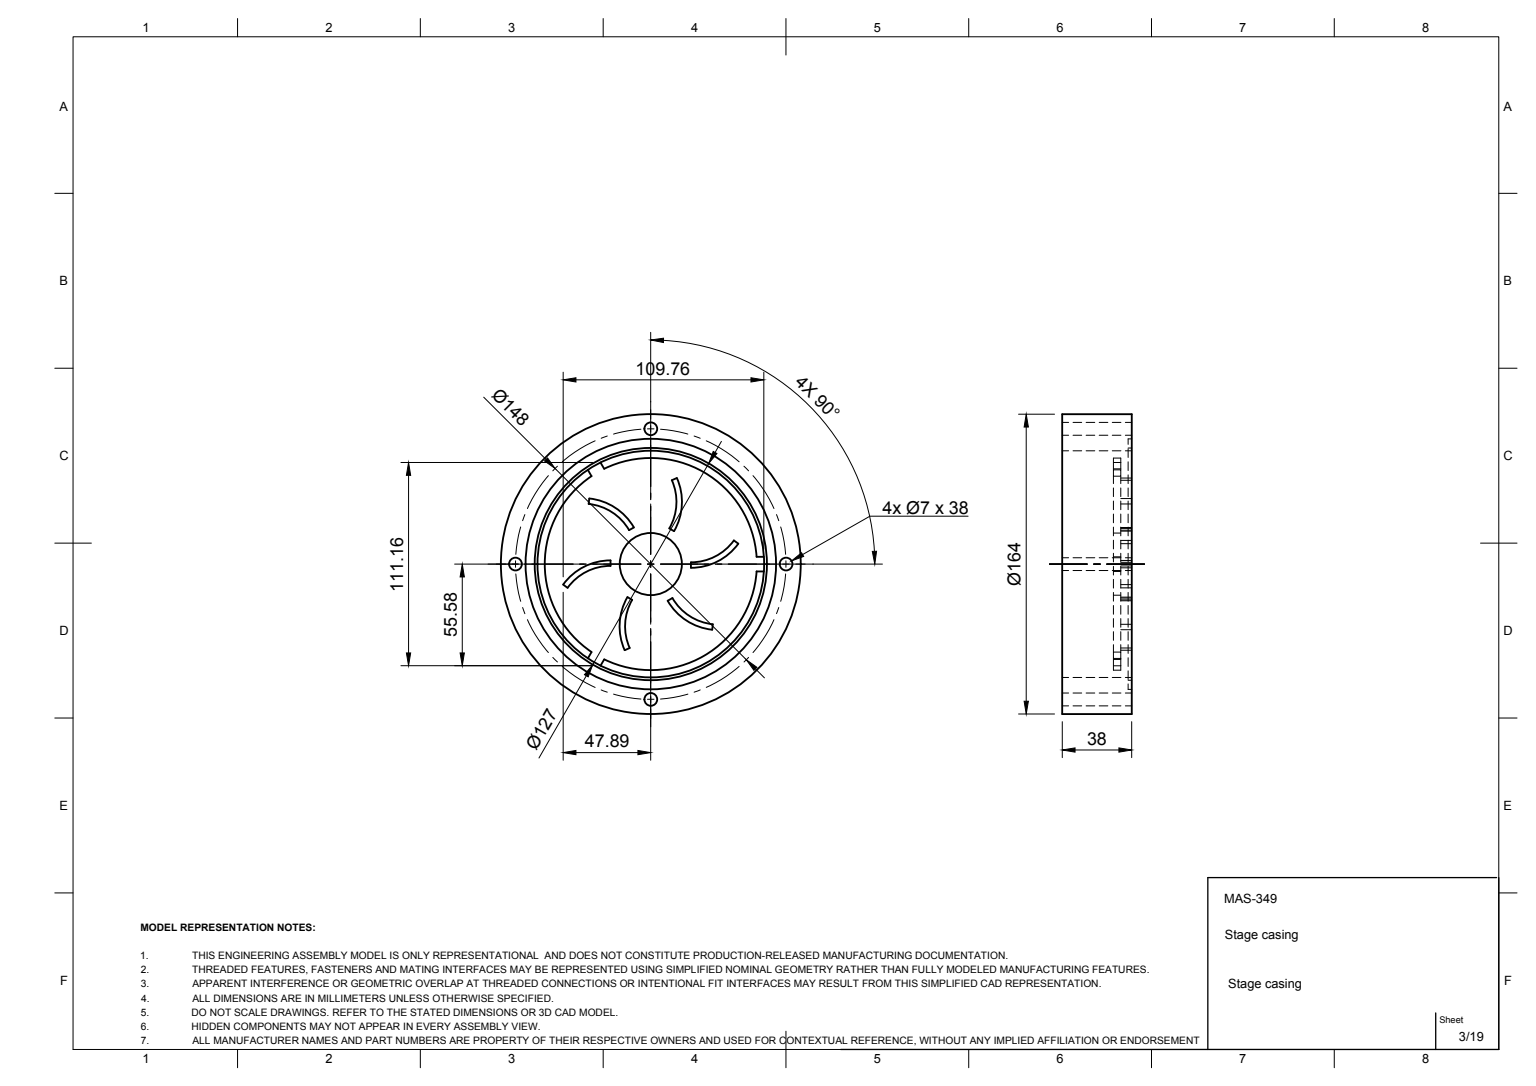
ISO-10303-21;
HEADER;
/* Generated by software containing ST-Developer
 * from STEP Tools, Inc. (www.steptools.com) 
 */

FILE_DESCRIPTION(
/* description */ ('Independent two-stage semi-open centrifugal-pump CAD. Shared impeller
s, open-machinable return casings, removable diaphragms, bronze wear/j
ournal rings, volume-preserving seal instances, retained keyed shaft, 
opposed mechanical face rings and partly threaded tie hardware. Native
 shaft rotation. Geometric topology/clearance only; flow/head/efficien
cy, pressure, cavitation, balance, preload, face loading and secondary
 seal fits/bonds, material/thermal/tolerance selection and life unassi
gned. External drive, coupling, anchors and piping bolts omitted.'),
/* implementation_level */ '2;1');

FILE_NAME(
/* name */ 'Stage casing.step',
/* time_stamp */ '2026-11-08T18:06:32-08:00',
/* author */ (''),
/* organization */ (''),
/* preprocessor_version */ 'ST-DEVELOPER v20.2',
/* originating_system */ 'Autodesk Translation Framework v15.17.0.0',
/* authorisation */ '');

FILE_SCHEMA (('AUTOMOTIVE_DESIGN { 1 0 10303 214 3 1 1 }'));
ENDSEC;

DATA;
#10=MECHANICAL_DESIGN_GEOMETRIC_PRESENTATION_REPRESENTATION('',(#393),#16687);
#355=SHAPE_REPRESENTATION_RELATIONSHIP('SRR','None',#16764,#374);
#374=ADVANCED_BREP_SHAPE_REPRESENTATION('',(#412),#16668);
#393=STYLED_ITEM('',(#16868),#412);
#412=MANIFOLD_SOLID_BREP('Body1',#6112);
#431=FACE_BOUND('',#1036,.T.);
#432=FACE_BOUND('',#1038,.T.);
#433=FACE_BOUND('',#1078,.T.);
#434=FACE_BOUND('',#1084,.T.);
#435=FACE_BOUND('',#1085,.T.);
#436=FACE_BOUND('',#1086,.T.);
#437=FACE_BOUND('',#1087,.T.);
#438=FACE_BOUND('',#1088,.T.);
#439=FACE_BOUND('',#1089,.T.);
#440=FACE_BOUND('',#1090,.T.);
#441=FACE_BOUND('',#1094,.T.);
#442=FACE_BOUND('',#1095,.T.);
#443=FACE_BOUND('',#1096,.T.);
#444=FACE_BOUND('',#1099,.T.);
#445=FACE_BOUND('',#1100,.T.);
#446=FACE_BOUND('',#1101,.T.);
#447=FACE_BOUND('',#1102,.T.);
#448=FACE_BOUND('',#1103,.T.);
#449=FACE_BOUND('',#1105,.T.);
#450=FACE_BOUND('',#1106,.T.);
#451=FACE_BOUND('',#1107,.T.);
#452=FACE_BOUND('',#1108,.T.);
#453=FACE_BOUND('',#1109,.T.);
#553=PLANE('',#6349);
#554=PLANE('',#6350);
#555=PLANE('',#6364);
#556=PLANE('',#6368);
#557=PLANE('',#6372);
#558=PLANE('',#6373);
#559=PLANE('',#6377);
#560=PLANE('',#6381);
#561=PLANE('',#6382);
#562=PLANE('',#6386);
#563=PLANE('',#6390);
#564=PLANE('',#6391);
#565=PLANE('',#6395);
#566=PLANE('',#6399);
#567=PLANE('',#6400);
#568=PLANE('',#6404);
#569=PLANE('',#6408);
#570=PLANE('',#6409);
#571=PLANE('',#6413);
#572=PLANE('',#6417);
#573=PLANE('',#6418);
#574=PLANE('',#6419);
#575=PLANE('',#6420);
#576=PLANE('',#6421);
#577=PLANE('',#6422);
#578=PLANE('',#6438);
#579=PLANE('',#6442);
#580=PLANE('',#6443);
#581=PLANE('',#6449);
#582=PLANE('',#6450);
#686=FACE_OUTER_BOUND('',#1033,.T.);
#687=FACE_OUTER_BOUND('',#1034,.T.);
#688=FACE_OUTER_BOUND('',#1035,.T.);
#689=FACE_OUTER_BOUND('',#1037,.T.);
#690=FACE_OUTER_BOUND('',#1039,.T.);
#691=FACE_OUTER_BOUND('',#1040,.T.);
#692=FACE_OUTER_BOUND('',#1041,.T.);
#693=FACE_OUTER_BOUND('',#1042,.T.);
#694=FACE_OUTER_BOUND('',#1043,.T.);
#695=FACE_OUTER_BOUND('',#1044,.T.);
#696=FACE_OUTER_BOUND('',#1045,.T.);
#697=FACE_OUTER_BOUND('',#1046,.T.);
#698=FACE_OUTER_BOUND('',#1047,.T.);
#699=FACE_OUTER_BOUND('',#1048,.T.);
#700=FACE_OUTER_BOUND('',#1049,.T.);
#701=FACE_OUTER_BOUND('',#1050,.T.);
#702=FACE_OUTER_BOUND('',#1051,.T.);
#703=FACE_OUTER_BOUND('',#1052,.T.);
#704=FACE_OUTER_BOUND('',#1053,.T.);
#705=FACE_OUTER_BOUND('',#1054,.T.);
#706=FACE_OUTER_BOUND('',#1055,.T.);
#707=FACE_OUTER_BOUND('',#1056,.T.);
#708=FACE_OUTER_BOUND('',#1057,.T.);
#709=FACE_OUTER_BOUND('',#1058,.T.);
#710=FACE_OUTER_BOUND('',#1059,.T.);
#711=FACE_OUTER_BOUND('',#1060,.T.);
#712=FACE_OUTER_BOUND('',#1061,.T.);
#713=FACE_OUTER_BOUND('',#1062,.T.);
#714=FACE_OUTER_BOUND('',#1063,.T.);
#715=FACE_OUTER_BOUND('',#1064,.T.);
#716=FACE_OUTER_BOUND('',#1065,.T.);
#717=FACE_OUTER_BOUND('',#1066,.T.);
#718=FACE_OUTER_BOUND('',#1067,.T.);
#719=FACE_OUTER_BOUND('',#1068,.T.);
#720=FACE_OUTER_BOUND('',#1069,.T.);
#721=FACE_OUTER_BOUND('',#1070,.T.);
#722=FACE_OUTER_BOUND('',#1071,.T.);
#723=FACE_OUTER_BOUND('',#1072,.T.);
#724=FACE_OUTER_BOUND('',#1073,.T.);
#725=FACE_OUTER_BOUND('',#1074,.T.);
#726=FACE_OUTER_BOUND('',#1075,.T.);
#727=FACE_OUTER_BOUND('',#1076,.T.);
#728=FACE_OUTER_BOUND('',#1077,.T.);
#729=FACE_OUTER_BOUND('',#1079,.T.);
#730=FACE_OUTER_BOUND('',#1080,.T.);
#731=FACE_OUTER_BOUND('',#1081,.T.);
#732=FACE_OUTER_BOUND('',#1082,.T.);
#733=FACE_OUTER_BOUND('',#1083,.T.);
#734=FACE_OUTER_BOUND('',#1091,.T.);
#735=FACE_OUTER_BOUND('',#1092,.T.);
#736=FACE_OUTER_BOUND('',#1093,.T.);
#737=FACE_OUTER_BOUND('',#1097,.T.);
#738=FACE_OUTER_BOUND('',#1098,.T.);
#739=FACE_OUTER_BOUND('',#1104,.T.);
#1033=EDGE_LOOP('',(#3891,#3892,#3893,#3894));
#1034=EDGE_LOOP('',(#3895,#3896,#3897,#3898));
#1035=EDGE_LOOP('',(#3899));
#1036=EDGE_LOOP('',(#3900));
#1037=EDGE_LOOP('',(#3901));
#1038=EDGE_LOOP('',(#3902));
#1039=EDGE_LOOP('',(#3903,#3904,#3905,#3906));
#1040=EDGE_LOOP('',(#3907,#3908,#3909,#3910));
#1041=EDGE_LOOP('',(#3911,#3912,#3913,#3914));
#1042=EDGE_LOOP('',(#3915,#3916,#3917,#3918));
#1043=EDGE_LOOP('',(#3919,#3920,#3921,#3922));
#1044=EDGE_LOOP('',(#3923,#3924,#3925,#3926));
#1045=EDGE_LOOP('',(#3927,#3928,#3929,#3930));
#1046=EDGE_LOOP('',(#3931,#3932,#3933,#3934));
#1047=EDGE_LOOP('',(#3935,#3936,#3937,#3938));
#1048=EDGE_LOOP('',(#3939,#3940,#3941,#3942));
#1049=EDGE_LOOP('',(#3943,#3944,#3945,#3946));
#1050=EDGE_LOOP('',(#3947,#3948,#3949,#3950));
#1051=EDGE_LOOP('',(#3951,#3952,#3953,#3954));
#1052=EDGE_LOOP('',(#3955,#3956,#3957,#3958));
#1053=EDGE_LOOP('',(#3959,#3960,#3961,#3962));
#1054=EDGE_LOOP('',(#3963,#3964,#3965,#3966));
#1055=EDGE_LOOP('',(#3967,#3968,#3969,#3970));
#1056=EDGE_LOOP('',(#3971,#3972,#3973,#3974));
#1057=EDGE_LOOP('',(#3975,#3976,#3977,#3978));
#1058=EDGE_LOOP('',(#3979,#3980,#3981,#3982));
#1059=EDGE_LOOP('',(#3983,#3984,#3985,#3986));
#1060=EDGE_LOOP('',(#3987,#3988,#3989,#3990));
#1061=EDGE_LOOP('',(#3991,#3992,#3993,#3994));
#1062=EDGE_LOOP('',(#3995,#3996,#3997,#3998));
#1063=EDGE_LOOP('',(#3999,#4000,#4001,#4002));
#1064=EDGE_LOOP('',(#4003,#4004,#4005,#4006));
#1065=EDGE_LOOP('',(#4007,#4008,#4009,#4010));
#1066=EDGE_LOOP('',(#4011,#4012,#4013,#4014));
#1067=EDGE_LOOP('',(#4015,#4016,#4017,#4018));
#1068=EDGE_LOOP('',(#4019,#4020,#4021,#4022));
#1069=EDGE_LOOP('',(#4023,#4024,#4025,#4026));
#1070=EDGE_LOOP('',(#4027,#4028,#4029,#4030));
#1071=EDGE_LOOP('',(#4031,#4032,#4033,#4034));
#1072=EDGE_LOOP('',(#4035,#4036,#4037,#4038));
#1073=EDGE_LOOP('',(#4039,#4040,#4041,#4042));
#1074=EDGE_LOOP('',(#4043,#4044,#4045,#4046));
#1075=EDGE_LOOP('',(#4047,#4048,#4049,#4050));
#1076=EDGE_LOOP('',(#4051,#4052,#4053,#4054));
#1077=EDGE_LOOP('',(#4055,#4056,#4057,#4058,#4059,#4060,#4061,#4062,#4063,
#4064,#4065,#4066));
#1078=EDGE_LOOP('',(#4067));
#1079=EDGE_LOOP('',(#4068,#4069,#4070,#4071));
#1080=EDGE_LOOP('',(#4072,#4073,#4074,#4075));
#1081=EDGE_LOOP('',(#4076,#4077,#4078,#4079));
#1082=EDGE_LOOP('',(#4080,#4081,#4082,#4083));
#1083=EDGE_LOOP('',(#4084,#4085,#4086,#4087,#4088,#4089,#4090,#4091,#4092,
#4093,#4094,#4095));
#1084=EDGE_LOOP('',(#4096));
#1085=EDGE_LOOP('',(#4097,#4098,#4099,#4100));
#1086=EDGE_LOOP('',(#4101,#4102,#4103,#4104));
#1087=EDGE_LOOP('',(#4105,#4106,#4107,#4108));
#1088=EDGE_LOOP('',(#4109,#4110,#4111,#4112));
#1089=EDGE_LOOP('',(#4113,#4114,#4115,#4116));
#1090=EDGE_LOOP('',(#4117,#4118,#4119,#4120));
#1091=EDGE_LOOP('',(#4121,#4122,#4123,#4124));
#1092=EDGE_LOOP('',(#4125,#4126,#4127,#4128));
#1093=EDGE_LOOP('',(#4129,#4130,#4131,#4132));
#1094=EDGE_LOOP('',(#4133,#4134,#4135,#4136));
#1095=EDGE_LOOP('',(#4137,#4138,#4139,#4140));
#1096=EDGE_LOOP('',(#4141,#4142,#4143,#4144));
#1097=EDGE_LOOP('',(#4145,#4146,#4147,#4148));
#1098=EDGE_LOOP('',(#4149));
#1099=EDGE_LOOP('',(#4150));
#1100=EDGE_LOOP('',(#4151));
#1101=EDGE_LOOP('',(#4152));
#1102=EDGE_LOOP('',(#4153));
#1103=EDGE_LOOP('',(#4154));
#1104=EDGE_LOOP('',(#4155));
#1105=EDGE_LOOP('',(#4156));
#1106=EDGE_LOOP('',(#4157));
#1107=EDGE_LOOP('',(#4158));
#1108=EDGE_LOOP('',(#4159));
#1109=EDGE_LOOP('',(#4160));
#1502=LINE('',#8657,#1871);
#1503=LINE('',#8663,#1872);
#1504=LINE('',#8673,#1873);
#1505=LINE('',#8679,#1874);
#1506=LINE('',#8685,#1875);
#1507=LINE('',#8691,#1876);
#1508=LINE('',#8696,#1877);
#1509=LINE('',#8698,#1878);
#1510=LINE('',#8700,#1879);
#1511=LINE('',#8701,#1880);
#1512=LINE('',#8707,#1881);
#1513=LINE('',#8710,#1882);
#1514=LINE('',#8712,#1883);
#1515=LINE('',#8713,#1884);
#1516=LINE('',#8721,#1885);
#1517=LINE('',#8723,#1886);
#1518=LINE('',#8725,#1887);
#1519=LINE('',#8726,#1888);
#1520=LINE('',#8732,#1889);
#1521=LINE('',#8735,#1890);
#1522=LINE('',#8737,#1891);
#1523=LINE('',#8738,#1892);
#1524=LINE('',#8746,#1893);
#1525=LINE('',#8748,#1894);
#1526=LINE('',#8750,#1895);
#1527=LINE('',#8751,#1896);
#1528=LINE('',#8757,#1897);
#1529=LINE('',#8760,#1898);
#1530=LINE('',#8762,#1899);
#1531=LINE('',#8763,#1900);
#1532=LINE('',#8771,#1901);
#1533=LINE('',#8773,#1902);
#1534=LINE('',#8775,#1903);
#1535=LINE('',#8776,#1904);
#1536=LINE('',#8782,#1905);
#1537=LINE('',#8785,#1906);
#1538=LINE('',#8787,#1907);
#1539=LINE('',#8788,#1908);
#1540=LINE('',#8796,#1909);
#1541=LINE('',#8798,#1910);
#1542=LINE('',#8800,#1911);
#1543=LINE('',#8801,#1912);
#1544=LINE('',#8807,#1913);
#1545=LINE('',#8810,#1914);
#1546=LINE('',#8812,#1915);
#1547=LINE('',#8813,#1916);
#1548=LINE('',#8821,#1917);
#1549=LINE('',#8823,#1918);
#1550=LINE('',#8825,#1919);
#1551=LINE('',#8826,#1920);
#1552=LINE('',#8832,#1921);
#1553=LINE('',#8835,#1922);
#1554=LINE('',#8837,#1923);
#1555=LINE('',#8838,#1924);
#1556=LINE('',#8846,#1925);
#1557=LINE('',#8848,#1926);
#1558=LINE('',#8850,#1927);
#1559=LINE('',#8851,#1928);
#1560=LINE('',#8855,#1929);
#1561=LINE('',#8857,#1930);
#1562=LINE('',#8859,#1931);
#1563=LINE('',#8860,#1932);
#1564=LINE('',#8864,#1933);
#1565=LINE('',#8866,#1934);
#1566=LINE('',#8868,#1935);
#1567=LINE('',#8869,#1936);
#1568=LINE('',#8873,#1937);
#1569=LINE('',#8875,#1938);
#1570=LINE('',#8877,#1939);
#1571=LINE('',#8878,#1940);
#1572=LINE('',#8885,#1941);
#1573=LINE('',#8889,#1942);
#1574=LINE('',#8897,#1943);
#1575=LINE('',#8902,#1944);
#1576=LINE('',#8907,#1945);
#1577=LINE('',#8910,#1946);
#1578=LINE('',#8913,#1947);
#1579=LINE('',#8917,#1948);
#1580=LINE('',#8919,#1949);
#1581=LINE('',#8922,#1950);
#1582=LINE('',#8928,#1951);
#1871=VECTOR('',#6996,6.35);
#1872=VECTOR('',#7003,6.85);
#1873=VECTOR('',#7016,0.35);
#1874=VECTOR('',#7023,0.35);
#1875=VECTOR('',#7030,0.35);
#1876=VECTOR('',#7037,0.35);
#1877=VECTOR('',#7042,1.);
#1878=VECTOR('',#7043,1.);
#1879=VECTOR('',#7044,1.);
#1880=VECTOR('',#7045,1.);
#1881=VECTOR('',#7052,1.);
#1882=VECTOR('',#7055,1.);
#1883=VECTOR('',#7056,1.);
#1884=VECTOR('',#7057,1.);
#1885=VECTOR('',#7068,1.);
#1886=VECTOR('',#7069,1.);
#1887=VECTOR('',#7070,1.);
#1888=VECTOR('',#7071,1.);
#1889=VECTOR('',#7078,1.);
#1890=VECTOR('',#7081,1.);
#1891=VECTOR('',#7082,1.);
#1892=VECTOR('',#7083,1.);
#1893=VECTOR('',#7094,1.);
#1894=VECTOR('',#7095,1.);
#1895=VECTOR('',#7096,1.);
#1896=VECTOR('',#7097,1.);
#1897=VECTOR('',#7104,1.);
#1898=VECTOR('',#7107,1.);
#1899=VECTOR('',#7108,1.);
#1900=VECTOR('',#7109,1.);
#1901=VECTOR('',#7120,1.);
#1902=VECTOR('',#7121,1.);
#1903=VECTOR('',#7122,1.);
#1904=VECTOR('',#7123,1.);
#1905=VECTOR('',#7130,1.);
#1906=VECTOR('',#7133,1.);
#1907=VECTOR('',#7134,1.);
#1908=VECTOR('',#7135,1.);
#1909=VECTOR('',#7146,1.);
#1910=VECTOR('',#7147,1.);
#1911=VECTOR('',#7148,1.);
#1912=VECTOR('',#7149,1.);
#1913=VECTOR('',#7156,1.);
#1914=VECTOR('',#7159,1.);
#1915=VECTOR('',#7160,1.);
#1916=VECTOR('',#7161,1.);
#1917=VECTOR('',#7172,1.);
#1918=VECTOR('',#7173,1.);
#1919=VECTOR('',#7174,1.);
#1920=VECTOR('',#7175,1.);
#1921=VECTOR('',#7182,1.);
#1922=VECTOR('',#7185,1.);
#1923=VECTOR('',#7186,1.);
#1924=VECTOR('',#7187,1.);
#1925=VECTOR('',#7198,1.);
#1926=VECTOR('',#7199,1.);
#1927=VECTOR('',#7200,1.);
#1928=VECTOR('',#7201,1.);
#1929=VECTOR('',#7204,1.);
#1930=VECTOR('',#7205,1.);
#1931=VECTOR('',#7206,1.);
#1932=VECTOR('',#7207,1.);
#1933=VECTOR('',#7210,1.);
#1934=VECTOR('',#7211,1.);
#1935=VECTOR('',#7212,1.);
#1936=VECTOR('',#7213,1.);
#1937=VECTOR('',#7216,1.);
#1938=VECTOR('',#7217,1.);
#1939=VECTOR('',#7218,1.);
#1940=VECTOR('',#7219,1.);
#1941=VECTOR('',#7228,1.);
#1942=VECTOR('',#7231,1.);
#1943=VECTOR('',#7242,1.);
#1944=VECTOR('',#7249,1.);
#1945=VECTOR('',#7256,1.7);
#1946=VECTOR('',#7259,1.);
#1947=VECTOR('',#7262,1.);
#1948=VECTOR('',#7269,1.);
#1949=VECTOR('',#7272,1.);
#1950=VECTOR('',#7275,6.2);
#1951=VECTOR('',#7282,8.2);
#2240=CIRCLE('',#6344,6.35);
#2241=CIRCLE('',#6345,6.35);
#2242=CIRCLE('',#6347,6.85);
#2243=CIRCLE('',#6348,6.85);
#2244=CIRCLE('',#6351,6.2);
#2245=CIRCLE('',#6353,0.35);
#2246=CIRCLE('',#6354,0.35);
#2247=CIRCLE('',#6356,0.35);
#2248=CIRCLE('',#6357,0.35);
#2249=CIRCLE('',#6359,0.35);
#2250=CIRCLE('',#6360,0.35);
#2251=CIRCLE('',#6362,0.35);
#2252=CIRCLE('',#6363,0.35);
#2253=CIRCLE('',#6366,2.9);
#2254=CIRCLE('',#6367,2.9);
#2255=CIRCLE('',#6370,3.2);
#2256=CIRCLE('',#6371,3.2);
#2257=CIRCLE('',#6375,2.9);
#2258=CIRCLE('',#6376,2.9);
#2259=CIRCLE('',#6379,3.2);
#2260=CIRCLE('',#6380,3.2);
#2261=CIRCLE('',#6384,2.9);
#2262=CIRCLE('',#6385,2.9);
#2263=CIRCLE('',#6388,3.2);
#2264=CIRCLE('',#6389,3.2);
#2265=CIRCLE('',#6393,2.9);
#2266=CIRCLE('',#6394,2.9);
#2267=CIRCLE('',#6397,3.2);
#2268=CIRCLE('',#6398,3.2);
#2269=CIRCLE('',#6402,2.9);
#2270=CIRCLE('',#6403,2.9);
#2271=CIRCLE('',#6406,3.2);
#2272=CIRCLE('',#6407,3.2);
#2273=CIRCLE('',#6411,2.9);
#2274=CIRCLE('',#6412,2.9);
#2275=CIRCLE('',#6415,3.2);
#2276=CIRCLE('',#6416,3.2);
#2277=CIRCLE('',#6423,5.8);
#2278=CIRCLE('',#6424,6.2);
#2279=CIRCLE('',#6425,5.8);
#2280=CIRCLE('',#6426,6.2);
#2281=CIRCLE('',#6427,5.8);
#2282=CIRCLE('',#6428,6.2);
#2283=CIRCLE('',#6429,1.7);
#2284=CIRCLE('',#6431,5.8);
#2285=CIRCLE('',#6433,5.8);
#2286=CIRCLE('',#6435,5.8);
#2287=CIRCLE('',#6437,1.7);
#2288=CIRCLE('',#6439,6.2);
#2289=CIRCLE('',#6440,6.2);
#2290=CIRCLE('',#6441,6.2);
#2291=CIRCLE('',#6445,6.2);
#2292=CIRCLE('',#6447,8.2);
#2293=CIRCLE('',#6448,8.2);
#2499=VERTEX_POINT('',#8654);
#2500=VERTEX_POINT('',#8656);
#2501=VERTEX_POINT('',#8660);
#2502=VERTEX_POINT('',#8662);
#2503=VERTEX_POINT('',#8667);
#2504=VERTEX_POINT('',#8670);
#2505=VERTEX_POINT('',#8672);
#2506=VERTEX_POINT('',#8676);
#2507=VERTEX_POINT('',#8678);
#2508=VERTEX_POINT('',#8682);
#2509=VERTEX_POINT('',#8684);
#2510=VERTEX_POINT('',#8688);
#2511=VERTEX_POINT('',#8690);
#2512=VERTEX_POINT('',#8694);
#2513=VERTEX_POINT('',#8695);
#2514=VERTEX_POINT('',#8697);
#2515=VERTEX_POINT('',#8699);
#2516=VERTEX_POINT('',#8703);
#2517=VERTEX_POINT('',#8705);
#2518=VERTEX_POINT('',#8709);
#2519=VERTEX_POINT('',#8711);
#2520=VERTEX_POINT('',#8719);
#2521=VERTEX_POINT('',#8720);
#2522=VERTEX_POINT('',#8722);
#2523=VERTEX_POINT('',#8724);
#2524=VERTEX_POINT('',#8728);
#2525=VERTEX_POINT('',#8730);
#2526=VERTEX_POINT('',#8734);
#2527=VERTEX_POINT('',#8736);
#2528=VERTEX_POINT('',#8744);
#2529=VERTEX_POINT('',#8745);
#2530=VERTEX_POINT('',#8747);
#2531=VERTEX_POINT('',#8749);
#2532=VERTEX_POINT('',#8753);
#2533=VERTEX_POINT('',#8755);
#2534=VERTEX_POINT('',#8759);
#2535=VERTEX_POINT('',#8761);
#2536=VERTEX_POINT('',#8769);
#2537=VERTEX_POINT('',#8770);
#2538=VERTEX_POINT('',#8772);
#2539=VERTEX_POINT('',#8774);
#2540=VERTEX_POINT('',#8778);
#2541=VERTEX_POINT('',#8780);
#2542=VERTEX_POINT('',#8784);
#2543=VERTEX_POINT('',#8786);
#2544=VERTEX_POINT('',#8794);
#2545=VERTEX_POINT('',#8795);
#2546=VERTEX_POINT('',#8797);
#2547=VERTEX_POINT('',#8799);
#2548=VERTEX_POINT('',#8803);
#2549=VERTEX_POINT('',#8805);
#2550=VERTEX_POINT('',#8809);
#2551=VERTEX_POINT('',#8811);
#2552=VERTEX_POINT('',#8819);
#2553=VERTEX_POINT('',#8820);
#2554=VERTEX_POINT('',#8822);
#2555=VERTEX_POINT('',#8824);
#2556=VERTEX_POINT('',#8828);
#2557=VERTEX_POINT('',#8830);
#2558=VERTEX_POINT('',#8834);
#2559=VERTEX_POINT('',#8836);
#2560=VERTEX_POINT('',#8844);
#2561=VERTEX_POINT('',#8845);
#2562=VERTEX_POINT('',#8847);
#2563=VERTEX_POINT('',#8849);
#2564=VERTEX_POINT('',#8853);
#2565=VERTEX_POINT('',#8854);
#2566=VERTEX_POINT('',#8856);
#2567=VERTEX_POINT('',#8858);
#2568=VERTEX_POINT('',#8862);
#2569=VERTEX_POINT('',#8863);
#2570=VERTEX_POINT('',#8865);
#2571=VERTEX_POINT('',#8867);
#2572=VERTEX_POINT('',#8871);
#2573=VERTEX_POINT('',#8872);
#2574=VERTEX_POINT('',#8874);
#2575=VERTEX_POINT('',#8876);
#2576=VERTEX_POINT('',#8882);
#2577=VERTEX_POINT('',#8884);
#2578=VERTEX_POINT('',#8886);
#2579=VERTEX_POINT('',#8888);
#2580=VERTEX_POINT('',#8892);
#2581=VERTEX_POINT('',#8895);
#2582=VERTEX_POINT('',#8901);
#2583=VERTEX_POINT('',#8905);
#2584=VERTEX_POINT('',#8909);
#2585=VERTEX_POINT('',#8911);
#2586=VERTEX_POINT('',#8921);
#2587=VERTEX_POINT('',#8925);
#2588=VERTEX_POINT('',#8927);
#3055=EDGE_CURVE('',#2499,#2499,#2240,.T.);
#3056=EDGE_CURVE('',#2499,#2500,#1502,.T.);
#3057=EDGE_CURVE('',#2500,#2500,#2241,.T.);
#3058=EDGE_CURVE('',#2501,#2501,#2242,.T.);
#3059=EDGE_CURVE('',#2501,#2502,#1503,.T.);
#3060=EDGE_CURVE('',#2502,#2502,#2243,.T.);
#3061=EDGE_CURVE('',#2503,#2503,#2244,.T.);
#3062=EDGE_CURVE('',#2504,#2504,#2245,.T.);
#3063=EDGE_CURVE('',#2504,#2505,#1504,.T.);
#3064=EDGE_CURVE('',#2505,#2505,#2246,.T.);
#3065=EDGE_CURVE('',#2506,#2506,#2247,.T.);
#3066=EDGE_CURVE('',#2506,#2507,#1505,.T.);
#3067=EDGE_CURVE('',#2507,#2507,#2248,.T.);
#3068=EDGE_CURVE('',#2508,#2508,#2249,.T.);
#3069=EDGE_CURVE('',#2508,#2509,#1506,.T.);
#3070=EDGE_CURVE('',#2509,#2509,#2250,.T.);
#3071=EDGE_CURVE('',#2510,#2510,#2251,.T.);
#3072=EDGE_CURVE('',#2510,#2511,#1507,.T.);
#3073=EDGE_CURVE('',#2511,#2511,#2252,.T.);
#3074=EDGE_CURVE('',#2512,#2513,#1508,.T.);
#3075=EDGE_CURVE('',#2512,#2514,#1509,.T.);
#3076=EDGE_CURVE('',#2515,#2514,#1510,.T.);
#3077=EDGE_CURVE('',#2513,#2515,#1511,.T.);
#3078=EDGE_CURVE('',#2513,#2516,#2253,.T.);
#3079=EDGE_CURVE('',#2517,#2515,#2254,.T.);
#3080=EDGE_CURVE('',#2516,#2517,#1512,.T.);
#3081=EDGE_CURVE('',#2516,#2518,#1513,.T.);
#3082=EDGE_CURVE('',#2519,#2517,#1514,.T.);
#3083=EDGE_CURVE('',#2518,#2519,#1515,.T.);
#3084=EDGE_CURVE('',#2518,#2512,#2255,.T.);
#3085=EDGE_CURVE('',#2514,#2519,#2256,.T.);
#3086=EDGE_CURVE('',#2520,#2521,#1516,.T.);
#3087=EDGE_CURVE('',#2520,#2522,#1517,.T.);
#3088=EDGE_CURVE('',#2523,#2522,#1518,.T.);
#3089=EDGE_CURVE('',#2521,#2523,#1519,.T.);
#3090=EDGE_CURVE('',#2521,#2524,#2257,.T.);
#3091=EDGE_CURVE('',#2525,#2523,#2258,.T.);
#3092=EDGE_CURVE('',#2524,#2525,#1520,.T.);
#3093=EDGE_CURVE('',#2524,#2526,#1521,.T.);
#3094=EDGE_CURVE('',#2527,#2525,#1522,.T.);
#3095=EDGE_CURVE('',#2526,#2527,#1523,.T.);
#3096=EDGE_CURVE('',#2526,#2520,#2259,.T.);
#3097=EDGE_CURVE('',#2522,#2527,#2260,.T.);
#3098=EDGE_CURVE('',#2528,#2529,#1524,.T.);
#3099=EDGE_CURVE('',#2528,#2530,#1525,.T.);
#3100=EDGE_CURVE('',#2531,#2530,#1526,.T.);
#3101=EDGE_CURVE('',#2529,#2531,#1527,.T.);
#3102=EDGE_CURVE('',#2529,#2532,#2261,.T.);
#3103=EDGE_CURVE('',#2533,#2531,#2262,.T.);
#3104=EDGE_CURVE('',#2532,#2533,#1528,.T.);
#3105=EDGE_CURVE('',#2532,#2534,#1529,.T.);
#3106=EDGE_CURVE('',#2535,#2533,#1530,.T.);
#3107=EDGE_CURVE('',#2534,#2535,#1531,.T.);
#3108=EDGE_CURVE('',#2534,#2528,#2263,.T.);
#3109=EDGE_CURVE('',#2530,#2535,#2264,.T.);
#3110=EDGE_CURVE('',#2536,#2537,#1532,.T.);
#3111=EDGE_CURVE('',#2536,#2538,#1533,.T.);
#3112=EDGE_CURVE('',#2539,#2538,#1534,.T.);
#3113=EDGE_CURVE('',#2537,#2539,#1535,.T.);
#3114=EDGE_CURVE('',#2537,#2540,#2265,.T.);
#3115=EDGE_CURVE('',#2541,#2539,#2266,.T.);
#3116=EDGE_CURVE('',#2540,#2541,#1536,.T.);
#3117=EDGE_CURVE('',#2540,#2542,#1537,.T.);
#3118=EDGE_CURVE('',#2543,#2541,#1538,.T.);
#3119=EDGE_CURVE('',#2542,#2543,#1539,.T.);
#3120=EDGE_CURVE('',#2542,#2536,#2267,.T.);
#3121=EDGE_CURVE('',#2538,#2543,#2268,.T.);
#3122=EDGE_CURVE('',#2544,#2545,#1540,.T.);
#3123=EDGE_CURVE('',#2544,#2546,#1541,.T.);
#3124=EDGE_CURVE('',#2547,#2546,#1542,.T.);
#3125=EDGE_CURVE('',#2545,#2547,#1543,.T.);
#3126=EDGE_CURVE('',#2545,#2548,#2269,.T.);
#3127=EDGE_CURVE('',#2549,#2547,#2270,.T.);
#3128=EDGE_CURVE('',#2548,#2549,#1544,.T.);
#3129=EDGE_CURVE('',#2548,#2550,#1545,.T.);
#3130=EDGE_CURVE('',#2551,#2549,#1546,.T.);
#3131=EDGE_CURVE('',#2550,#2551,#1547,.T.);
#3132=EDGE_CURVE('',#2550,#2544,#2271,.T.);
#3133=EDGE_CURVE('',#2546,#2551,#2272,.T.);
#3134=EDGE_CURVE('',#2552,#2553,#1548,.T.);
#3135=EDGE_CURVE('',#2552,#2554,#1549,.T.);
#3136=EDGE_CURVE('',#2555,#2554,#1550,.T.);
#3137=EDGE_CURVE('',#2553,#2555,#1551,.T.);
#3138=EDGE_CURVE('',#2553,#2556,#2273,.T.);
#3139=EDGE_CURVE('',#2557,#2555,#2274,.T.);
#3140=EDGE_CURVE('',#2556,#2557,#1552,.T.);
#3141=EDGE_CURVE('',#2556,#2558,#1553,.T.);
#3142=EDGE_CURVE('',#2559,#2557,#1554,.T.);
#3143=EDGE_CURVE('',#2558,#2559,#1555,.T.);
#3144=EDGE_CURVE('',#2558,#2552,#2275,.T.);
#3145=EDGE_CURVE('',#2554,#2559,#2276,.T.);
#3146=EDGE_CURVE('',#2560,#2561,#1556,.T.);
#3147=EDGE_CURVE('',#2562,#2560,#1557,.T.);
#3148=EDGE_CURVE('',#2563,#2562,#1558,.T.);
#3149=EDGE_CURVE('',#2563,#2561,#1559,.T.);
#3150=EDGE_CURVE('',#2564,#2565,#1560,.T.);
#3151=EDGE_CURVE('',#2564,#2566,#1561,.T.);
#3152=EDGE_CURVE('',#2567,#2566,#1562,.T.);
#3153=EDGE_CURVE('',#2565,#2567,#1563,.T.);
#3154=EDGE_CURVE('',#2568,#2569,#1564,.T.);
#3155=EDGE_CURVE('',#2570,#2568,#1565,.T.);
#3156=EDGE_CURVE('',#2571,#2570,#1566,.T.);
#3157=EDGE_CURVE('',#2571,#2569,#1567,.T.);
#3158=EDGE_CURVE('',#2572,#2573,#1568,.T.);
#3159=EDGE_CURVE('',#2572,#2574,#1569,.T.);
#3160=EDGE_CURVE('',#2575,#2574,#1570,.T.);
#3161=EDGE_CURVE('',#2573,#2575,#1571,.T.);
#3162=EDGE_CURVE('',#2569,#2564,#2277,.T.);
#3163=EDGE_CURVE('',#2574,#2571,#2278,.T.);
#3164=EDGE_CURVE('',#2576,#2572,#2279,.T.);
#3165=EDGE_CURVE('',#2577,#2576,#1572,.T.);
#3166=EDGE_CURVE('',#2578,#2577,#2280,.T.);
#3167=EDGE_CURVE('',#2579,#2578,#1573,.T.);
#3168=EDGE_CURVE('',#2561,#2579,#2281,.T.);
#3169=EDGE_CURVE('',#2566,#2563,#2282,.T.);
#3170=EDGE_CURVE('',#2580,#2580,#2283,.T.);
#3171=EDGE_CURVE('',#2581,#2573,#2284,.T.);
#3172=EDGE_CURVE('',#2576,#2581,#1574,.T.);
#3173=EDGE_CURVE('',#2568,#2565,#2285,.T.);
#3174=EDGE_CURVE('',#2582,#2579,#1575,.T.);
#3175=EDGE_CURVE('',#2560,#2582,#2286,.T.);
#3176=EDGE_CURVE('',#2583,#2583,#2287,.T.);
#3177=EDGE_CURVE('',#2583,#2580,#1576,.T.);
#3178=EDGE_CURVE('',#2582,#2584,#1577,.T.);
#3179=EDGE_CURVE('',#2585,#2584,#2288,.T.);
#3180=EDGE_CURVE('',#2585,#2581,#1578,.T.);
#3181=EDGE_CURVE('',#2570,#2575,#2289,.T.);
#3182=EDGE_CURVE('',#2562,#2567,#2290,.T.);
#3183=EDGE_CURVE('',#2584,#2578,#1579,.T.);
#3184=EDGE_CURVE('',#2577,#2585,#1580,.T.);
#3185=EDGE_CURVE('',#2503,#2586,#1581,.T.);
#3186=EDGE_CURVE('',#2586,#2586,#2291,.T.);
#3187=EDGE_CURVE('',#2587,#2587,#2292,.T.);
#3188=EDGE_CURVE('',#2587,#2588,#1582,.T.);
#3189=EDGE_CURVE('',#2588,#2588,#2293,.T.);
#3891=ORIENTED_EDGE('',*,*,#3055,.F.);
#3892=ORIENTED_EDGE('',*,*,#3056,.T.);
#3893=ORIENTED_EDGE('',*,*,#3057,.T.);
#3894=ORIENTED_EDGE('',*,*,#3056,.F.);
#3895=ORIENTED_EDGE('',*,*,#3058,.F.);
#3896=ORIENTED_EDGE('',*,*,#3059,.T.);
#3897=ORIENTED_EDGE('',*,*,#3060,.T.);
#3898=ORIENTED_EDGE('',*,*,#3059,.F.);
#3899=ORIENTED_EDGE('',*,*,#3060,.F.);
#3900=ORIENTED_EDGE('',*,*,#3057,.F.);
#3901=ORIENTED_EDGE('',*,*,#3055,.T.);
#3902=ORIENTED_EDGE('',*,*,#3061,.T.);
#3903=ORIENTED_EDGE('',*,*,#3062,.F.);
#3904=ORIENTED_EDGE('',*,*,#3063,.T.);
#3905=ORIENTED_EDGE('',*,*,#3064,.F.);
#3906=ORIENTED_EDGE('',*,*,#3063,.F.);
#3907=ORIENTED_EDGE('',*,*,#3065,.F.);
#3908=ORIENTED_EDGE('',*,*,#3066,.T.);
#3909=ORIENTED_EDGE('',*,*,#3067,.F.);
#3910=ORIENTED_EDGE('',*,*,#3066,.F.);
#3911=ORIENTED_EDGE('',*,*,#3068,.F.);
#3912=ORIENTED_EDGE('',*,*,#3069,.T.);
#3913=ORIENTED_EDGE('',*,*,#3070,.F.);
#3914=ORIENTED_EDGE('',*,*,#3069,.F.);
#3915=ORIENTED_EDGE('',*,*,#3071,.F.);
#3916=ORIENTED_EDGE('',*,*,#3072,.T.);
#3917=ORIENTED_EDGE('',*,*,#3073,.F.);
#3918=ORIENTED_EDGE('',*,*,#3072,.F.);
#3919=ORIENTED_EDGE('',*,*,#3074,.F.);
#3920=ORIENTED_EDGE('',*,*,#3075,.T.);
#3921=ORIENTED_EDGE('',*,*,#3076,.F.);
#3922=ORIENTED_EDGE('',*,*,#3077,.F.);
#3923=ORIENTED_EDGE('',*,*,#3078,.F.);
#3924=ORIENTED_EDGE('',*,*,#3077,.T.);
#3925=ORIENTED_EDGE('',*,*,#3079,.F.);
#3926=ORIENTED_EDGE('',*,*,#3080,.F.);
#3927=ORIENTED_EDGE('',*,*,#3081,.F.);
#3928=ORIENTED_EDGE('',*,*,#3080,.T.);
#3929=ORIENTED_EDGE('',*,*,#3082,.F.);
#3930=ORIENTED_EDGE('',*,*,#3083,.F.);
#3931=ORIENTED_EDGE('',*,*,#3084,.F.);
#3932=ORIENTED_EDGE('',*,*,#3083,.T.);
#3933=ORIENTED_EDGE('',*,*,#3085,.F.);
#3934=ORIENTED_EDGE('',*,*,#3075,.F.);
#3935=ORIENTED_EDGE('',*,*,#3085,.T.);
#3936=ORIENTED_EDGE('',*,*,#3082,.T.);
#3937=ORIENTED_EDGE('',*,*,#3079,.T.);
#3938=ORIENTED_EDGE('',*,*,#3076,.T.);
#3939=ORIENTED_EDGE('',*,*,#3086,.F.);
#3940=ORIENTED_EDGE('',*,*,#3087,.T.);
#3941=ORIENTED_EDGE('',*,*,#3088,.F.);
#3942=ORIENTED_EDGE('',*,*,#3089,.F.);
#3943=ORIENTED_EDGE('',*,*,#3090,.F.);
#3944=ORIENTED_EDGE('',*,*,#3089,.T.);
#3945=ORIENTED_EDGE('',*,*,#3091,.F.);
#3946=ORIENTED_EDGE('',*,*,#3092,.F.);
#3947=ORIENTED_EDGE('',*,*,#3093,.F.);
#3948=ORIENTED_EDGE('',*,*,#3092,.T.);
#3949=ORIENTED_EDGE('',*,*,#3094,.F.);
#3950=ORIENTED_EDGE('',*,*,#3095,.F.);
#3951=ORIENTED_EDGE('',*,*,#3096,.F.);
#3952=ORIENTED_EDGE('',*,*,#3095,.T.);
#3953=ORIENTED_EDGE('',*,*,#3097,.F.);
#3954=ORIENTED_EDGE('',*,*,#3087,.F.);
#3955=ORIENTED_EDGE('',*,*,#3097,.T.);
#3956=ORIENTED_EDGE('',*,*,#3094,.T.);
#3957=ORIENTED_EDGE('',*,*,#3091,.T.);
#3958=ORIENTED_EDGE('',*,*,#3088,.T.);
#3959=ORIENTED_EDGE('',*,*,#3098,.F.);
#3960=ORIENTED_EDGE('',*,*,#3099,.T.);
#3961=ORIENTED_EDGE('',*,*,#3100,.F.);
#3962=ORIENTED_EDGE('',*,*,#3101,.F.);
#3963=ORIENTED_EDGE('',*,*,#3102,.F.);
#3964=ORIENTED_EDGE('',*,*,#3101,.T.);
#3965=ORIENTED_EDGE('',*,*,#3103,.F.);
#3966=ORIENTED_EDGE('',*,*,#3104,.F.);
#3967=ORIENTED_EDGE('',*,*,#3105,.F.);
#3968=ORIENTED_EDGE('',*,*,#3104,.T.);
#3969=ORIENTED_EDGE('',*,*,#3106,.F.);
#3970=ORIENTED_EDGE('',*,*,#3107,.F.);
#3971=ORIENTED_EDGE('',*,*,#3108,.F.);
#3972=ORIENTED_EDGE('',*,*,#3107,.T.);
#3973=ORIENTED_EDGE('',*,*,#3109,.F.);
#3974=ORIENTED_EDGE('',*,*,#3099,.F.);
#3975=ORIENTED_EDGE('',*,*,#3109,.T.);
#3976=ORIENTED_EDGE('',*,*,#3106,.T.);
#3977=ORIENTED_EDGE('',*,*,#3103,.T.);
#3978=ORIENTED_EDGE('',*,*,#3100,.T.);
#3979=ORIENTED_EDGE('',*,*,#3110,.F.);
#3980=ORIENTED_EDGE('',*,*,#3111,.T.);
#3981=ORIENTED_EDGE('',*,*,#3112,.F.);
#3982=ORIENTED_EDGE('',*,*,#3113,.F.);
#3983=ORIENTED_EDGE('',*,*,#3114,.F.);
#3984=ORIENTED_EDGE('',*,*,#3113,.T.);
#3985=ORIENTED_EDGE('',*,*,#3115,.F.);
#3986=ORIENTED_EDGE('',*,*,#3116,.F.);
#3987=ORIENTED_EDGE('',*,*,#3117,.F.);
#3988=ORIENTED_EDGE('',*,*,#3116,.T.);
#3989=ORIENTED_EDGE('',*,*,#3118,.F.);
#3990=ORIENTED_EDGE('',*,*,#3119,.F.);
#3991=ORIENTED_EDGE('',*,*,#3120,.F.);
#3992=ORIENTED_EDGE('',*,*,#3119,.T.);
#3993=ORIENTED_EDGE('',*,*,#3121,.F.);
#3994=ORIENTED_EDGE('',*,*,#3111,.F.);
#3995=ORIENTED_EDGE('',*,*,#3121,.T.);
#3996=ORIENTED_EDGE('',*,*,#3118,.T.);
#3997=ORIENTED_EDGE('',*,*,#3115,.T.);
#3998=ORIENTED_EDGE('',*,*,#3112,.T.);
#3999=ORIENTED_EDGE('',*,*,#3122,.F.);
#4000=ORIENTED_EDGE('',*,*,#3123,.T.);
#4001=ORIENTED_EDGE('',*,*,#3124,.F.);
#4002=ORIENTED_EDGE('',*,*,#3125,.F.);
#4003=ORIENTED_EDGE('',*,*,#3126,.F.);
#4004=ORIENTED_EDGE('',*,*,#3125,.T.);
#4005=ORIENTED_EDGE('',*,*,#3127,.F.);
#4006=ORIENTED_EDGE('',*,*,#3128,.F.);
#4007=ORIENTED_EDGE('',*,*,#3129,.F.);
#4008=ORIENTED_EDGE('',*,*,#3128,.T.);
#4009=ORIENTED_EDGE('',*,*,#3130,.F.);
#4010=ORIENTED_EDGE('',*,*,#3131,.F.);
#4011=ORIENTED_EDGE('',*,*,#3132,.F.);
#4012=ORIENTED_EDGE('',*,*,#3131,.T.);
#4013=ORIENTED_EDGE('',*,*,#3133,.F.);
#4014=ORIENTED_EDGE('',*,*,#3123,.F.);
#4015=ORIENTED_EDGE('',*,*,#3133,.T.);
#4016=ORIENTED_EDGE('',*,*,#3130,.T.);
#4017=ORIENTED_EDGE('',*,*,#3127,.T.);
#4018=ORIENTED_EDGE('',*,*,#3124,.T.);
#4019=ORIENTED_EDGE('',*,*,#3134,.F.);
#4020=ORIENTED_EDGE('',*,*,#3135,.T.);
#4021=ORIENTED_EDGE('',*,*,#3136,.F.);
#4022=ORIENTED_EDGE('',*,*,#3137,.F.);
#4023=ORIENTED_EDGE('',*,*,#3138,.F.);
#4024=ORIENTED_EDGE('',*,*,#3137,.T.);
#4025=ORIENTED_EDGE('',*,*,#3139,.F.);
#4026=ORIENTED_EDGE('',*,*,#3140,.F.);
#4027=ORIENTED_EDGE('',*,*,#3141,.F.);
#4028=ORIENTED_EDGE('',*,*,#3140,.T.);
#4029=ORIENTED_EDGE('',*,*,#3142,.F.);
#4030=ORIENTED_EDGE('',*,*,#3143,.F.);
#4031=ORIENTED_EDGE('',*,*,#3144,.F.);
#4032=ORIENTED_EDGE('',*,*,#3143,.T.);
#4033=ORIENTED_EDGE('',*,*,#3145,.F.);
#4034=ORIENTED_EDGE('',*,*,#3135,.F.);
#4035=ORIENTED_EDGE('',*,*,#3145,.T.);
#4036=ORIENTED_EDGE('',*,*,#3142,.T.);
#4037=ORIENTED_EDGE('',*,*,#3139,.T.);
#4038=ORIENTED_EDGE('',*,*,#3136,.T.);
#4039=ORIENTED_EDGE('',*,*,#3146,.F.);
#4040=ORIENTED_EDGE('',*,*,#3147,.F.);
#4041=ORIENTED_EDGE('',*,*,#3148,.F.);
#4042=ORIENTED_EDGE('',*,*,#3149,.T.);
#4043=ORIENTED_EDGE('',*,*,#3150,.F.);
#4044=ORIENTED_EDGE('',*,*,#3151,.T.);
#4045=ORIENTED_EDGE('',*,*,#3152,.F.);
#4046=ORIENTED_EDGE('',*,*,#3153,.F.);
#4047=ORIENTED_EDGE('',*,*,#3154,.F.);
#4048=ORIENTED_EDGE('',*,*,#3155,.F.);
#4049=ORIENTED_EDGE('',*,*,#3156,.F.);
#4050=ORIENTED_EDGE('',*,*,#3157,.T.);
#4051=ORIENTED_EDGE('',*,*,#3158,.F.);
#4052=ORIENTED_EDGE('',*,*,#3159,.T.);
#4053=ORIENTED_EDGE('',*,*,#3160,.F.);
#4054=ORIENTED_EDGE('',*,*,#3161,.F.);
#4055=ORIENTED_EDGE('',*,*,#3162,.F.);
#4056=ORIENTED_EDGE('',*,*,#3157,.F.);
#4057=ORIENTED_EDGE('',*,*,#3163,.F.);
#4058=ORIENTED_EDGE('',*,*,#3159,.F.);
#4059=ORIENTED_EDGE('',*,*,#3164,.F.);
#4060=ORIENTED_EDGE('',*,*,#3165,.F.);
#4061=ORIENTED_EDGE('',*,*,#3166,.F.);
#4062=ORIENTED_EDGE('',*,*,#3167,.F.);
#4063=ORIENTED_EDGE('',*,*,#3168,.F.);
#4064=ORIENTED_EDGE('',*,*,#3149,.F.);
#4065=ORIENTED_EDGE('',*,*,#3169,.F.);
#4066=ORIENTED_EDGE('',*,*,#3151,.F.);
#4067=ORIENTED_EDGE('',*,*,#3170,.F.);
#4068=ORIENTED_EDGE('',*,*,#3158,.T.);
#4069=ORIENTED_EDGE('',*,*,#3171,.F.);
#4070=ORIENTED_EDGE('',*,*,#3172,.F.);
#4071=ORIENTED_EDGE('',*,*,#3164,.T.);
#4072=ORIENTED_EDGE('',*,*,#3150,.T.);
#4073=ORIENTED_EDGE('',*,*,#3173,.F.);
#4074=ORIENTED_EDGE('',*,*,#3154,.T.);
#4075=ORIENTED_EDGE('',*,*,#3162,.T.);
#4076=ORIENTED_EDGE('',*,*,#3146,.T.);
#4077=ORIENTED_EDGE('',*,*,#3168,.T.);
#4078=ORIENTED_EDGE('',*,*,#3174,.F.);
#4079=ORIENTED_EDGE('',*,*,#3175,.F.);
#4080=ORIENTED_EDGE('',*,*,#3176,.F.);
#4081=ORIENTED_EDGE('',*,*,#3177,.T.);
#4082=ORIENTED_EDGE('',*,*,#3170,.T.);
#4083=ORIENTED_EDGE('',*,*,#3177,.F.);
#4084=ORIENTED_EDGE('',*,*,#3175,.T.);
#4085=ORIENTED_EDGE('',*,*,#3178,.T.);
#4086=ORIENTED_EDGE('',*,*,#3179,.F.);
#4087=ORIENTED_EDGE('',*,*,#3180,.T.);
#4088=ORIENTED_EDGE('',*,*,#3171,.T.);
#4089=ORIENTED_EDGE('',*,*,#3161,.T.);
#4090=ORIENTED_EDGE('',*,*,#3181,.F.);
#4091=ORIENTED_EDGE('',*,*,#3155,.T.);
#4092=ORIENTED_EDGE('',*,*,#3173,.T.);
#4093=ORIENTED_EDGE('',*,*,#3153,.T.);
#4094=ORIENTED_EDGE('',*,*,#3182,.F.);
#4095=ORIENTED_EDGE('',*,*,#3147,.T.);
#4096=ORIENTED_EDGE('',*,*,#3176,.T.);
#4097=ORIENTED_EDGE('',*,*,#3134,.T.);
#4098=ORIENTED_EDGE('',*,*,#3138,.T.);
#4099=ORIENTED_EDGE('',*,*,#3141,.T.);
#4100=ORIENTED_EDGE('',*,*,#3144,.T.);
#4101=ORIENTED_EDGE('',*,*,#3122,.T.);
#4102=ORIENTED_EDGE('',*,*,#3126,.T.);
#4103=ORIENTED_EDGE('',*,*,#3129,.T.);
#4104=ORIENTED_EDGE('',*,*,#3132,.T.);
#4105=ORIENTED_EDGE('',*,*,#3110,.T.);
#4106=ORIENTED_EDGE('',*,*,#3114,.T.);
#4107=ORIENTED_EDGE('',*,*,#3117,.T.);
#4108=ORIENTED_EDGE('',*,*,#3120,.T.);
#4109=ORIENTED_EDGE('',*,*,#3098,.T.);
#4110=ORIENTED_EDGE('',*,*,#3102,.T.);
#4111=ORIENTED_EDGE('',*,*,#3105,.T.);
#4112=ORIENTED_EDGE('',*,*,#3108,.T.);
#4113=ORIENTED_EDGE('',*,*,#3086,.T.);
#4114=ORIENTED_EDGE('',*,*,#3090,.T.);
#4115=ORIENTED_EDGE('',*,*,#3093,.T.);
#4116=ORIENTED_EDGE('',*,*,#3096,.T.);
#4117=ORIENTED_EDGE('',*,*,#3074,.T.);
#4118=ORIENTED_EDGE('',*,*,#3078,.T.);
#4119=ORIENTED_EDGE('',*,*,#3081,.T.);
#4120=ORIENTED_EDGE('',*,*,#3084,.T.);
#4121=ORIENTED_EDGE('',*,*,#3174,.T.);
#4122=ORIENTED_EDGE('',*,*,#3167,.T.);
#4123=ORIENTED_EDGE('',*,*,#3183,.F.);
#4124=ORIENTED_EDGE('',*,*,#3178,.F.);
#4125=ORIENTED_EDGE('',*,*,#3172,.T.);
#4126=ORIENTED_EDGE('',*,*,#3180,.F.);
#4127=ORIENTED_EDGE('',*,*,#3184,.F.);
#4128=ORIENTED_EDGE('',*,*,#3165,.T.);
#4129=ORIENTED_EDGE('',*,*,#3061,.F.);
#4130=ORIENTED_EDGE('',*,*,#3185,.T.);
#4131=ORIENTED_EDGE('',*,*,#3186,.T.);
#4132=ORIENTED_EDGE('',*,*,#3185,.F.);
#4133=ORIENTED_EDGE('',*,*,#3152,.T.);
#4134=ORIENTED_EDGE('',*,*,#3169,.T.);
#4135=ORIENTED_EDGE('',*,*,#3148,.T.);
#4136=ORIENTED_EDGE('',*,*,#3182,.T.);
#4137=ORIENTED_EDGE('',*,*,#3160,.T.);
#4138=ORIENTED_EDGE('',*,*,#3163,.T.);
#4139=ORIENTED_EDGE('',*,*,#3156,.T.);
#4140=ORIENTED_EDGE('',*,*,#3181,.T.);
#4141=ORIENTED_EDGE('',*,*,#3183,.T.);
#4142=ORIENTED_EDGE('',*,*,#3166,.T.);
#4143=ORIENTED_EDGE('',*,*,#3184,.T.);
#4144=ORIENTED_EDGE('',*,*,#3179,.T.);
#4145=ORIENTED_EDGE('',*,*,#3187,.F.);
#4146=ORIENTED_EDGE('',*,*,#3188,.T.);
#4147=ORIENTED_EDGE('',*,*,#3189,.T.);
#4148=ORIENTED_EDGE('',*,*,#3188,.F.);
#4149=ORIENTED_EDGE('',*,*,#3187,.T.);
#4150=ORIENTED_EDGE('',*,*,#3062,.T.);
#4151=ORIENTED_EDGE('',*,*,#3065,.T.);
#4152=ORIENTED_EDGE('',*,*,#3068,.T.);
#4153=ORIENTED_EDGE('',*,*,#3071,.T.);
#4154=ORIENTED_EDGE('',*,*,#3058,.T.);
#4155=ORIENTED_EDGE('',*,*,#3189,.F.);
#4156=ORIENTED_EDGE('',*,*,#3186,.F.);
#4157=ORIENTED_EDGE('',*,*,#3073,.T.);
#4158=ORIENTED_EDGE('',*,*,#3070,.T.);
#4159=ORIENTED_EDGE('',*,*,#3067,.T.);
#4160=ORIENTED_EDGE('',*,*,#3064,.T.);
#5563=CYLINDRICAL_SURFACE('',#6343,6.35);
#5564=CYLINDRICAL_SURFACE('',#6346,6.85);
#5565=CYLINDRICAL_SURFACE('',#6352,0.35);
#5566=CYLINDRICAL_SURFACE('',#6355,0.35);
#5567=CYLINDRICAL_SURFACE('',#6358,0.35);
#5568=CYLINDRICAL_SURFACE('',#6361,0.35);
#5569=CYLINDRICAL_SURFACE('',#6365,2.9);
#5570=CYLINDRICAL_SURFACE('',#6369,3.2);
#5571=CYLINDRICAL_SURFACE('',#6374,2.9);
#5572=CYLINDRICAL_SURFACE('',#6378,3.2);
#5573=CYLINDRICAL_SURFACE('',#6383,2.9);
#5574=CYLINDRICAL_SURFACE('',#6387,3.2);
#5575=CYLINDRICAL_SURFACE('',#6392,2.9);
#5576=CYLINDRICAL_SURFACE('',#6396,3.2);
#5577=CYLINDRICAL_SURFACE('',#6401,2.9);
#5578=CYLINDRICAL_SURFACE('',#6405,3.2);
#5579=CYLINDRICAL_SURFACE('',#6410,2.9);
#5580=CYLINDRICAL_SURFACE('',#6414,3.2);
#5581=CYLINDRICAL_SURFACE('',#6430,5.8);
#5582=CYLINDRICAL_SURFACE('',#6432,5.8);
#5583=CYLINDRICAL_SURFACE('',#6434,5.8);
#5584=CYLINDRICAL_SURFACE('',#6436,1.7);
#5585=CYLINDRICAL_SURFACE('',#6444,6.2);
#5586=CYLINDRICAL_SURFACE('',#6446,8.2);
#5765=ADVANCED_FACE('',(#686),#5563,.T.);
#5766=ADVANCED_FACE('',(#687),#5564,.F.);
#5767=ADVANCED_FACE('',(#688,#431),#553,.T.);
#5768=ADVANCED_FACE('',(#689,#432),#554,.T.);
#5769=ADVANCED_FACE('',(#690),#5565,.F.);
#5770=ADVANCED_FACE('',(#691),#5566,.F.);
#5771=ADVANCED_FACE('',(#692),#5567,.F.);
#5772=ADVANCED_FACE('',(#693),#5568,.F.);
#5773=ADVANCED_FACE('',(#694),#555,.T.);
#5774=ADVANCED_FACE('',(#695),#5569,.F.);
#5775=ADVANCED_FACE('',(#696),#556,.T.);
#5776=ADVANCED_FACE('',(#697),#5570,.T.);
#5777=ADVANCED_FACE('',(#698),#557,.T.);
#5778=ADVANCED_FACE('',(#699),#558,.T.);
#5779=ADVANCED_FACE('',(#700),#5571,.F.);
#5780=ADVANCED_FACE('',(#701),#559,.T.);
#5781=ADVANCED_FACE('',(#702),#5572,.T.);
#5782=ADVANCED_FACE('',(#703),#560,.T.);
#5783=ADVANCED_FACE('',(#704),#561,.T.);
#5784=ADVANCED_FACE('',(#705),#5573,.F.);
#5785=ADVANCED_FACE('',(#706),#562,.T.);
#5786=ADVANCED_FACE('',(#707),#5574,.T.);
#5787=ADVANCED_FACE('',(#708),#563,.T.);
#5788=ADVANCED_FACE('',(#709),#564,.T.);
#5789=ADVANCED_FACE('',(#710),#5575,.F.);
#5790=ADVANCED_FACE('',(#711),#565,.T.);
#5791=ADVANCED_FACE('',(#712),#5576,.T.);
#5792=ADVANCED_FACE('',(#713),#566,.T.);
#5793=ADVANCED_FACE('',(#714),#567,.T.);
#5794=ADVANCED_FACE('',(#715),#5577,.F.);
#5795=ADVANCED_FACE('',(#716),#568,.T.);
#5796=ADVANCED_FACE('',(#717),#5578,.T.);
#5797=ADVANCED_FACE('',(#718),#569,.T.);
#5798=ADVANCED_FACE('',(#719),#570,.T.);
#5799=ADVANCED_FACE('',(#720),#5579,.F.);
#5800=ADVANCED_FACE('',(#721),#571,.T.);
#5801=ADVANCED_FACE('',(#722),#5580,.T.);
#5802=ADVANCED_FACE('',(#723),#572,.T.);
#5803=ADVANCED_FACE('',(#724),#573,.T.);
#5804=ADVANCED_FACE('',(#725),#574,.T.);
#5805=ADVANCED_FACE('',(#726),#575,.T.);
#5806=ADVANCED_FACE('',(#727),#576,.T.);
#5807=ADVANCED_FACE('',(#728,#433),#577,.F.);
#5808=ADVANCED_FACE('',(#729),#5581,.T.);
#5809=ADVANCED_FACE('',(#730),#5582,.T.);
#5810=ADVANCED_FACE('',(#731),#5583,.T.);
#5811=ADVANCED_FACE('',(#732),#5584,.F.);
#5812=ADVANCED_FACE('',(#733,#434,#435,#436,#437,#438,#439,#440),#578,.T.);
#5813=ADVANCED_FACE('',(#734),#579,.T.);
#5814=ADVANCED_FACE('',(#735),#580,.T.);
#5815=ADVANCED_FACE('',(#736,#441,#442,#443),#5585,.F.);
#5816=ADVANCED_FACE('',(#737),#5586,.T.);
#5817=ADVANCED_FACE('',(#738,#444,#445,#446,#447,#448),#581,.T.);
#5818=ADVANCED_FACE('',(#739,#449,#450,#451,#452,#453),#582,.F.);
#6112=CLOSED_SHELL('',(#5765,#5766,#5767,#5768,#5769,#5770,#5771,#5772,
#5773,#5774,#5775,#5776,#5777,#5778,#5779,#5780,#5781,#5782,#5783,#5784,
#5785,#5786,#5787,#5788,#5789,#5790,#5791,#5792,#5793,#5794,#5795,#5796,
#5797,#5798,#5799,#5800,#5801,#5802,#5803,#5804,#5805,#5806,#5807,#5808,
#5809,#5810,#5811,#5812,#5813,#5814,#5815,#5816,#5817,#5818));
#6342=AXIS2_PLACEMENT_3D('',#8652,#6990,#6991);
#6343=AXIS2_PLACEMENT_3D('',#8653,#6992,#6993);
#6344=AXIS2_PLACEMENT_3D('',#8655,#6994,#6995);
#6345=AXIS2_PLACEMENT_3D('',#8658,#6997,#6998);
#6346=AXIS2_PLACEMENT_3D('',#8659,#6999,#7000);
#6347=AXIS2_PLACEMENT_3D('',#8661,#7001,#7002);
#6348=AXIS2_PLACEMENT_3D('',#8664,#7004,#7005);
#6349=AXIS2_PLACEMENT_3D('',#8665,#7006,#7007);
#6350=AXIS2_PLACEMENT_3D('',#8666,#7008,#7009);
#6351=AXIS2_PLACEMENT_3D('',#8668,#7010,#7011);
#6352=AXIS2_PLACEMENT_3D('',#8669,#7012,#7013);
#6353=AXIS2_PLACEMENT_3D('',#8671,#7014,#7015);
#6354=AXIS2_PLACEMENT_3D('',#8674,#7017,#7018);
#6355=AXIS2_PLACEMENT_3D('',#8675,#7019,#7020);
#6356=AXIS2_PLACEMENT_3D('',#8677,#7021,#7022);
#6357=AXIS2_PLACEMENT_3D('',#8680,#7024,#7025);
#6358=AXIS2_PLACEMENT_3D('',#8681,#7026,#7027);
#6359=AXIS2_PLACEMENT_3D('',#8683,#7028,#7029);
#6360=AXIS2_PLACEMENT_3D('',#8686,#7031,#7032);
#6361=AXIS2_PLACEMENT_3D('',#8687,#7033,#7034);
#6362=AXIS2_PLACEMENT_3D('',#8689,#7035,#7036);
#6363=AXIS2_PLACEMENT_3D('',#8692,#7038,#7039);
#6364=AXIS2_PLACEMENT_3D('',#8693,#7040,#7041);
#6365=AXIS2_PLACEMENT_3D('',#8702,#7046,#7047);
#6366=AXIS2_PLACEMENT_3D('',#8704,#7048,#7049);
#6367=AXIS2_PLACEMENT_3D('',#8706,#7050,#7051);
#6368=AXIS2_PLACEMENT_3D('',#8708,#7053,#7054);
#6369=AXIS2_PLACEMENT_3D('',#8714,#7058,#7059);
#6370=AXIS2_PLACEMENT_3D('',#8715,#7060,#7061);
#6371=AXIS2_PLACEMENT_3D('',#8716,#7062,#7063);
#6372=AXIS2_PLACEMENT_3D('',#8717,#7064,#7065);
#6373=AXIS2_PLACEMENT_3D('',#8718,#7066,#7067);
#6374=AXIS2_PLACEMENT_3D('',#8727,#7072,#7073);
#6375=AXIS2_PLACEMENT_3D('',#8729,#7074,#7075);
#6376=AXIS2_PLACEMENT_3D('',#8731,#7076,#7077);
#6377=AXIS2_PLACEMENT_3D('',#8733,#7079,#7080);
#6378=AXIS2_PLACEMENT_3D('',#8739,#7084,#7085);
#6379=AXIS2_PLACEMENT_3D('',#8740,#7086,#7087);
#6380=AXIS2_PLACEMENT_3D('',#8741,#7088,#7089);
#6381=AXIS2_PLACEMENT_3D('',#8742,#7090,#7091);
#6382=AXIS2_PLACEMENT_3D('',#8743,#7092,#7093);
#6383=AXIS2_PLACEMENT_3D('',#8752,#7098,#7099);
#6384=AXIS2_PLACEMENT_3D('',#8754,#7100,#7101);
#6385=AXIS2_PLACEMENT_3D('',#8756,#7102,#7103);
#6386=AXIS2_PLACEMENT_3D('',#8758,#7105,#7106);
#6387=AXIS2_PLACEMENT_3D('',#8764,#7110,#7111);
#6388=AXIS2_PLACEMENT_3D('',#8765,#7112,#7113);
#6389=AXIS2_PLACEMENT_3D('',#8766,#7114,#7115);
#6390=AXIS2_PLACEMENT_3D('',#8767,#7116,#7117);
#6391=AXIS2_PLACEMENT_3D('',#8768,#7118,#7119);
#6392=AXIS2_PLACEMENT_3D('',#8777,#7124,#7125);
#6393=AXIS2_PLACEMENT_3D('',#8779,#7126,#7127);
#6394=AXIS2_PLACEMENT_3D('',#8781,#7128,#7129);
#6395=AXIS2_PLACEMENT_3D('',#8783,#7131,#7132);
#6396=AXIS2_PLACEMENT_3D('',#8789,#7136,#7137);
#6397=AXIS2_PLACEMENT_3D('',#8790,#7138,#7139);
#6398=AXIS2_PLACEMENT_3D('',#8791,#7140,#7141);
#6399=AXIS2_PLACEMENT_3D('',#8792,#7142,#7143);
#6400=AXIS2_PLACEMENT_3D('',#8793,#7144,#7145);
#6401=AXIS2_PLACEMENT_3D('',#8802,#7150,#7151);
#6402=AXIS2_PLACEMENT_3D('',#8804,#7152,#7153);
#6403=AXIS2_PLACEMENT_3D('',#8806,#7154,#7155);
#6404=AXIS2_PLACEMENT_3D('',#8808,#7157,#7158);
#6405=AXIS2_PLACEMENT_3D('',#8814,#7162,#7163);
#6406=AXIS2_PLACEMENT_3D('',#8815,#7164,#7165);
#6407=AXIS2_PLACEMENT_3D('',#8816,#7166,#7167);
#6408=AXIS2_PLACEMENT_3D('',#8817,#7168,#7169);
#6409=AXIS2_PLACEMENT_3D('',#8818,#7170,#7171);
#6410=AXIS2_PLACEMENT_3D('',#8827,#7176,#7177);
#6411=AXIS2_PLACEMENT_3D('',#8829,#7178,#7179);
#6412=AXIS2_PLACEMENT_3D('',#8831,#7180,#7181);
#6413=AXIS2_PLACEMENT_3D('',#8833,#7183,#7184);
#6414=AXIS2_PLACEMENT_3D('',#8839,#7188,#7189);
#6415=AXIS2_PLACEMENT_3D('',#8840,#7190,#7191);
#6416=AXIS2_PLACEMENT_3D('',#8841,#7192,#7193);
#6417=AXIS2_PLACEMENT_3D('',#8842,#7194,#7195);
#6418=AXIS2_PLACEMENT_3D('',#8843,#7196,#7197);
#6419=AXIS2_PLACEMENT_3D('',#8852,#7202,#7203);
#6420=AXIS2_PLACEMENT_3D('',#8861,#7208,#7209);
#6421=AXIS2_PLACEMENT_3D('',#8870,#7214,#7215);
#6422=AXIS2_PLACEMENT_3D('',#8879,#7220,#7221);
#6423=AXIS2_PLACEMENT_3D('',#8880,#7222,#7223);
#6424=AXIS2_PLACEMENT_3D('',#8881,#7224,#7225);
#6425=AXIS2_PLACEMENT_3D('',#8883,#7226,#7227);
#6426=AXIS2_PLACEMENT_3D('',#8887,#7229,#7230);
#6427=AXIS2_PLACEMENT_3D('',#8890,#7232,#7233);
#6428=AXIS2_PLACEMENT_3D('',#8891,#7234,#7235);
#6429=AXIS2_PLACEMENT_3D('',#8893,#7236,#7237);
#6430=AXIS2_PLACEMENT_3D('',#8894,#7238,#7239);
#6431=AXIS2_PLACEMENT_3D('',#8896,#7240,#7241);
#6432=AXIS2_PLACEMENT_3D('',#8898,#7243,#7244);
#6433=AXIS2_PLACEMENT_3D('',#8899,#7245,#7246);
#6434=AXIS2_PLACEMENT_3D('',#8900,#7247,#7248);
#6435=AXIS2_PLACEMENT_3D('',#8903,#7250,#7251);
#6436=AXIS2_PLACEMENT_3D('',#8904,#7252,#7253);
#6437=AXIS2_PLACEMENT_3D('',#8906,#7254,#7255);
#6438=AXIS2_PLACEMENT_3D('',#8908,#7257,#7258);
#6439=AXIS2_PLACEMENT_3D('',#8912,#7260,#7261);
#6440=AXIS2_PLACEMENT_3D('',#8914,#7263,#7264);
#6441=AXIS2_PLACEMENT_3D('',#8915,#7265,#7266);
#6442=AXIS2_PLACEMENT_3D('',#8916,#7267,#7268);
#6443=AXIS2_PLACEMENT_3D('',#8918,#7270,#7271);
#6444=AXIS2_PLACEMENT_3D('',#8920,#7273,#7274);
#6445=AXIS2_PLACEMENT_3D('',#8923,#7276,#7277);
#6446=AXIS2_PLACEMENT_3D('',#8924,#7278,#7279);
#6447=AXIS2_PLACEMENT_3D('',#8926,#7280,#7281);
#6448=AXIS2_PLACEMENT_3D('',#8929,#7283,#7284);
#6449=AXIS2_PLACEMENT_3D('',#8930,#7285,#7286);
#6450=AXIS2_PLACEMENT_3D('',#8931,#7287,#7288);
#6990=DIRECTION('axis',(0.,0.,1.));
#6991=DIRECTION('refdir',(1.,0.,0.));
#6992=DIRECTION('center_axis',(0.,0.,-1.));
#6993=DIRECTION('ref_axis',(1.,0.,0.));
#6994=DIRECTION('center_axis',(0.,0.,1.));
#6995=DIRECTION('ref_axis',(1.,0.,0.));
#6996=DIRECTION('',(0.,0.,-1.));
#6997=DIRECTION('center_axis',(0.,0.,1.));
#6998=DIRECTION('ref_axis',(1.,0.,0.));
#6999=DIRECTION('center_axis',(0.,0.,-1.));
#7000=DIRECTION('ref_axis',(1.,0.,0.));
#7001=DIRECTION('center_axis',(0.,0.,-1.));
#7002=DIRECTION('ref_axis',(1.,0.,0.));
#7003=DIRECTION('',(0.,0.,-1.));
#7004=DIRECTION('center_axis',(0.,0.,-1.));
#7005=DIRECTION('ref_axis',(1.,0.,0.));
#7006=DIRECTION('center_axis',(0.,0.,1.));
#7007=DIRECTION('ref_axis',(1.,0.,0.));
#7008=DIRECTION('center_axis',(0.,0.,1.));
#7009=DIRECTION('ref_axis',(1.,0.,0.));
#7010=DIRECTION('center_axis',(0.,0.,-1.));
#7011=DIRECTION('ref_axis',(1.,0.,0.));
#7012=DIRECTION('center_axis',(0.,0.,-1.));
#7013=DIRECTION('ref_axis',(1.,0.,0.));
#7014=DIRECTION('center_axis',(0.,0.,-1.));
#7015=DIRECTION('ref_axis',(1.,0.,0.));
#7016=DIRECTION('',(0.,0.,-1.));
#7017=DIRECTION('center_axis',(0.,0.,1.));
#7018=DIRECTION('ref_axis',(1.,0.,0.));
#7019=DIRECTION('center_axis',(0.,0.,-1.));
#7020=DIRECTION('ref_axis',(1.,0.,0.));
#7021=DIRECTION('center_axis',(0.,0.,-1.));
#7022=DIRECTION('ref_axis',(1.,0.,0.));
#7023=DIRECTION('',(0.,0.,-1.));
#7024=DIRECTION('center_axis',(0.,0.,1.));
#7025=DIRECTION('ref_axis',(1.,0.,0.));
#7026=DIRECTION('center_axis',(0.,0.,-1.));
#7027=DIRECTION('ref_axis',(1.,0.,0.));
#7028=DIRECTION('center_axis',(0.,0.,-1.));
#7029=DIRECTION('ref_axis',(1.,0.,0.));
#7030=DIRECTION('',(0.,0.,-1.));
#7031=DIRECTION('center_axis',(0.,0.,1.));
#7032=DIRECTION('ref_axis',(1.,0.,0.));
#7033=DIRECTION('center_axis',(0.,0.,-1.));
#7034=DIRECTION('ref_axis',(1.,0.,0.));
#7035=DIRECTION('center_axis',(0.,0.,-1.));
#7036=DIRECTION('ref_axis',(1.,0.,0.));
#7037=DIRECTION('',(0.,0.,-1.));
#7038=DIRECTION('center_axis',(0.,0.,1.));
#7039=DIRECTION('ref_axis',(1.,0.,0.));
#7040=DIRECTION('center_axis',(-0.499999999999999,0.866025403784439,0.));
#7041=DIRECTION('ref_axis',(-0.866025403784439,-0.499999999999999,0.));
#7042=DIRECTION('',(0.866025403784439,0.499999999999999,0.));
#7043=DIRECTION('',(0.,0.,1.));
#7044=DIRECTION('',(-0.866025403784439,-0.499999999999999,0.));
#7045=DIRECTION('',(0.,0.,1.));
#7046=DIRECTION('center_axis',(0.,0.,1.));
#7047=DIRECTION('ref_axis',(-0.866025403784439,-0.499999999999999,0.));
#7048=DIRECTION('center_axis',(0.,0.,1.));
#7049=DIRECTION('ref_axis',(-0.866025403784439,-0.499999999999999,0.));
#7050=DIRECTION('center_axis',(0.,0.,-1.));
#7051=DIRECTION('ref_axis',(-0.866025403784439,-0.499999999999999,0.));
#7052=DIRECTION('',(0.,0.,1.));
#7053=DIRECTION('center_axis',(0.994521895368273,-0.104528463267654,0.));
#7054=DIRECTION('ref_axis',(0.104528463267654,0.994521895368273,0.));
#7055=DIRECTION('',(-0.104528463267654,-0.994521895368273,0.));
#7056=DIRECTION('',(0.104528463267654,0.994521895368273,0.));
#7057=DIRECTION('',(0.,0.,1.));
#7058=DIRECTION('center_axis',(0.,0.,1.));
#7059=DIRECTION('ref_axis',(-0.866025403784439,-0.499999999999999,0.));
#7060=DIRECTION('center_axis',(0.,0.,-1.));
#7061=DIRECTION('ref_axis',(-0.866025403784439,-0.499999999999999,0.));
#7062=DIRECTION('center_axis',(0.,0.,1.));
#7063=DIRECTION('ref_axis',(-0.866025403784439,-0.499999999999999,0.));
#7064=DIRECTION('center_axis',(0.,0.,1.));
#7065=DIRECTION('ref_axis',(0.499999999999999,-0.866025403784439,0.));
#7066=DIRECTION('center_axis',(0.5,0.866025403784438,0.));
#7067=DIRECTION('ref_axis',(-0.866025403784438,0.5,0.));
#7068=DIRECTION('',(0.866025403784438,-0.5,0.));
#7069=DIRECTION('',(0.,0.,1.));
#7070=DIRECTION('',(-0.866025403784438,0.5,0.));
#7071=DIRECTION('',(0.,0.,1.));
#7072=DIRECTION('center_axis',(0.,0.,1.));
#7073=DIRECTION('ref_axis',(-0.866025403784438,0.5,0.));
#7074=DIRECTION('center_axis',(0.,0.,1.));
#7075=DIRECTION('ref_axis',(-0.866025403784438,0.5,0.));
#7076=DIRECTION('center_axis',(0.,0.,-1.));
#7077=DIRECTION('ref_axis',(-0.866025403784438,0.5,0.));
#7078=DIRECTION('',(0.,0.,1.));
#7079=DIRECTION('center_axis',(0.4067366430758,-0.913545457642601,0.));
#7080=DIRECTION('ref_axis',(0.913545457642601,0.4067366430758,0.));
#7081=DIRECTION('',(-0.913545457642601,-0.4067366430758,0.));
#7082=DIRECTION('',(0.913545457642601,0.4067366430758,0.));
#7083=DIRECTION('',(0.,0.,1.));
#7084=DIRECTION('center_axis',(0.,0.,1.));
#7085=DIRECTION('ref_axis',(-0.866025403784438,0.5,0.));
#7086=DIRECTION('center_axis',(0.,0.,-1.));
#7087=DIRECTION('ref_axis',(-0.866025403784438,0.5,0.));
#7088=DIRECTION('center_axis',(0.,0.,1.));
#7089=DIRECTION('ref_axis',(-0.866025403784438,0.5,0.));
#7090=DIRECTION('center_axis',(0.,0.,1.));
#7091=DIRECTION('ref_axis',(-0.5,-0.866025403784438,0.));
#7092=DIRECTION('center_axis',(1.,-1.66533453693773E-16,0.));
#7093=DIRECTION('ref_axis',(1.66533453693773E-16,1.,0.));
#7094=DIRECTION('',(-1.66533453693773E-16,-1.,0.));
#7095=DIRECTION('',(0.,0.,1.));
#7096=DIRECTION('',(1.66533453693773E-16,1.,0.));
#7097=DIRECTION('',(0.,0.,1.));
#7098=DIRECTION('center_axis',(0.,0.,1.));
#7099=DIRECTION('ref_axis',(1.53134210293125E-16,1.,0.));
#7100=DIRECTION('center_axis',(0.,0.,1.));
#7101=DIRECTION('ref_axis',(1.53134210293125E-16,1.,0.));
#7102=DIRECTION('center_axis',(0.,0.,-1.));
#7103=DIRECTION('ref_axis',(1.53134210293125E-16,1.,0.));
#7104=DIRECTION('',(0.,0.,1.));
#7105=DIRECTION('center_axis',(-0.587785252292473,-0.809016994374947,0.));
#7106=DIRECTION('ref_axis',(0.809016994374947,-0.587785252292473,0.));
#7107=DIRECTION('',(-0.809016994374947,0.587785252292473,0.));
#7108=DIRECTION('',(0.809016994374947,-0.587785252292473,0.));
#7109=DIRECTION('',(0.,0.,1.));
#7110=DIRECTION('center_axis',(0.,0.,1.));
#7111=DIRECTION('ref_axis',(-6.93889390390723E-17,1.,0.));
#7112=DIRECTION('center_axis',(0.,0.,-1.));
#7113=DIRECTION('ref_axis',(-6.93889390390723E-17,1.,0.));
#7114=DIRECTION('center_axis',(0.,0.,1.));
#7115=DIRECTION('ref_axis',(-6.93889390390723E-17,1.,0.));
#7116=DIRECTION('center_axis',(0.,0.,1.));
#7117=DIRECTION('ref_axis',(-1.,1.66533453693773E-16,0.));
#7118=DIRECTION('center_axis',(0.5,-0.866025403784439,0.));
#7119=DIRECTION('ref_axis',(0.866025403784439,0.5,0.));
#7120=DIRECTION('',(-0.866025403784439,-0.5,0.));
#7121=DIRECTION('',(0.,0.,1.));
#7122=DIRECTION('',(0.866025403784439,0.5,0.));
#7123=DIRECTION('',(0.,0.,1.));
#7124=DIRECTION('center_axis',(0.,0.,1.));
#7125=DIRECTION('ref_axis',(0.866025403784439,0.5,0.));
#7126=DIRECTION('center_axis',(0.,0.,1.));
#7127=DIRECTION('ref_axis',(0.866025403784439,0.5,0.));
#7128=DIRECTION('center_axis',(0.,0.,-1.));
#7129=DIRECTION('ref_axis',(0.866025403784439,0.5,0.));
#7130=DIRECTION('',(0.,0.,1.));
#7131=DIRECTION('center_axis',(-0.994521895368273,0.104528463267654,0.));
#7132=DIRECTION('ref_axis',(-0.104528463267654,-0.994521895368273,0.));
#7133=DIRECTION('',(0.104528463267654,0.994521895368273,0.));
#7134=DIRECTION('',(-0.104528463267654,-0.994521895368273,0.));
#7135=DIRECTION('',(0.,0.,1.));
#7136=DIRECTION('center_axis',(0.,0.,1.));
#7137=DIRECTION('ref_axis',(0.866025403784439,0.5,0.));
#7138=DIRECTION('center_axis',(0.,0.,-1.));
#7139=DIRECTION('ref_axis',(0.866025403784439,0.5,0.));
#7140=DIRECTION('center_axis',(0.,0.,1.));
#7141=DIRECTION('ref_axis',(0.866025403784439,0.5,0.));
#7142=DIRECTION('center_axis',(0.,0.,1.));
#7143=DIRECTION('ref_axis',(-0.5,0.866025403784439,0.));
#7144=DIRECTION('center_axis',(-0.5,-0.866025403784439,0.));
#7145=DIRECTION('ref_axis',(0.866025403784439,-0.5,0.));
#7146=DIRECTION('',(-0.866025403784439,0.5,0.));
#7147=DIRECTION('',(0.,0.,1.));
#7148=DIRECTION('',(0.866025403784439,-0.5,0.));
#7149=DIRECTION('',(0.,0.,1.));
#7150=DIRECTION('center_axis',(0.,0.,1.));
#7151=DIRECTION('ref_axis',(0.866025403784439,-0.5,0.));
#7152=DIRECTION('center_axis',(0.,0.,1.));
#7153=DIRECTION('ref_axis',(0.866025403784439,-0.5,0.));
#7154=DIRECTION('center_axis',(0.,0.,-1.));
#7155=DIRECTION('ref_axis',(0.866025403784439,-0.5,0.));
#7156=DIRECTION('',(0.,0.,1.));
#7157=DIRECTION('center_axis',(-0.4067366430758,0.913545457642601,0.));
#7158=DIRECTION('ref_axis',(-0.913545457642601,-0.4067366430758,0.));
#7159=DIRECTION('',(0.913545457642601,0.4067366430758,0.));
#7160=DIRECTION('',(-0.913545457642601,-0.4067366430758,0.));
#7161=DIRECTION('',(0.,0.,1.));
#7162=DIRECTION('center_axis',(0.,0.,1.));
#7163=DIRECTION('ref_axis',(0.866025403784439,-0.5,0.));
#7164=DIRECTION('center_axis',(0.,0.,-1.));
#7165=DIRECTION('ref_axis',(0.866025403784439,-0.5,0.));
#7166=DIRECTION('center_axis',(0.,0.,1.));
#7167=DIRECTION('ref_axis',(0.866025403784439,-0.5,0.));
#7168=DIRECTION('center_axis',(0.,0.,1.));
#7169=DIRECTION('ref_axis',(0.5,0.866025403784439,0.));
#7170=DIRECTION('center_axis',(-1.,0.,0.));
#7171=DIRECTION('ref_axis',(0.,-1.,0.));
#7172=DIRECTION('',(0.,1.,0.));
#7173=DIRECTION('',(0.,0.,1.));
#7174=DIRECTION('',(0.,-1.,0.));
#7175=DIRECTION('',(0.,0.,1.));
#7176=DIRECTION('center_axis',(0.,0.,1.));
#7177=DIRECTION('ref_axis',(0.,-1.,0.));
#7178=DIRECTION('center_axis',(0.,0.,1.));
#7179=DIRECTION('ref_axis',(0.,-1.,0.));
#7180=DIRECTION('center_axis',(0.,0.,-1.));
#7181=DIRECTION('ref_axis',(0.,-1.,0.));
#7182=DIRECTION('',(0.,0.,1.));
#7183=DIRECTION('center_axis',(0.587785252292473,0.809016994374947,0.));
#7184=DIRECTION('ref_axis',(-0.809016994374947,0.587785252292473,0.));
#7185=DIRECTION('',(0.809016994374947,-0.587785252292473,0.));
#7186=DIRECTION('',(-0.809016994374947,0.587785252292473,0.));
#7187=DIRECTION('',(0.,0.,1.));
#7188=DIRECTION('center_axis',(0.,0.,1.));
#7189=DIRECTION('ref_axis',(1.38777878078145E-16,-1.,0.));
#7190=DIRECTION('center_axis',(0.,0.,-1.));
#7191=DIRECTION('ref_axis',(1.38777878078145E-16,-1.,0.));
#7192=DIRECTION('center_axis',(0.,0.,1.));
#7193=DIRECTION('ref_axis',(1.38777878078145E-16,-1.,0.));
#7194=DIRECTION('center_axis',(0.,0.,1.));
#7195=DIRECTION('ref_axis',(1.,0.,0.));
#7196=DIRECTION('center_axis',(0.866025403784438,-0.5,0.));
#7197=DIRECTION('ref_axis',(0.5,0.866025403784438,0.));
#7198=DIRECTION('',(0.,0.,-1.));
#7199=DIRECTION('',(0.5,0.866025403784438,0.));
#7200=DIRECTION('',(0.,0.,1.));
#7201=DIRECTION('',(0.5,0.866025403784438,0.));
#7202=DIRECTION('center_axis',(-0.866025403784438,0.5,0.));
#7203=DIRECTION('ref_axis',(-0.5,-0.866025403784438,0.));
#7204=DIRECTION('',(0.,0.,1.));
#7205=DIRECTION('',(-0.5,-0.866025403784438,0.));
#7206=DIRECTION('',(0.,0.,-1.));
#7207=DIRECTION('',(-0.5,-0.866025403784438,0.));
#7208=DIRECTION('center_axis',(-0.866025403784439,-0.5,0.));
#7209=DIRECTION('ref_axis',(0.5,-0.866025403784439,0.));
#7210=DIRECTION('',(0.,0.,-1.));
#7211=DIRECTION('',(0.5,-0.866025403784439,0.));
#7212=DIRECTION('',(0.,0.,1.));
#7213=DIRECTION('',(0.5,-0.866025403784439,0.));
#7214=DIRECTION('center_axis',(0.866025403784439,0.5,0.));
#7215=DIRECTION('ref_axis',(-0.5,0.866025403784439,0.));
#7216=DIRECTION('',(0.,0.,1.));
#7217=DIRECTION('',(-0.5,0.866025403784439,0.));
#7218=DIRECTION('',(0.,0.,-1.));
#7219=DIRECTION('',(-0.5,0.866025403784439,0.));
#7220=DIRECTION('center_axis',(0.,0.,1.));
#7221=DIRECTION('ref_axis',(1.,0.,0.));
#7222=DIRECTION('center_axis',(0.,0.,1.));
#7223=DIRECTION('ref_axis',(1.,0.,0.));
#7224=DIRECTION('center_axis',(0.,0.,1.));
#7225=DIRECTION('ref_axis',(1.,0.,0.));
#7226=DIRECTION('center_axis',(0.,0.,1.));
#7227=DIRECTION('ref_axis',(1.,0.,0.));
#7228=DIRECTION('',(-1.,0.,0.));
#7229=DIRECTION('center_axis',(0.,0.,1.));
#7230=DIRECTION('ref_axis',(1.,0.,0.));
#7231=DIRECTION('',(1.,0.,0.));
#7232=DIRECTION('center_axis',(0.,0.,1.));
#7233=DIRECTION('ref_axis',(1.,0.,0.));
#7234=DIRECTION('center_axis',(0.,0.,1.));
#7235=DIRECTION('ref_axis',(1.,0.,0.));
#7236=DIRECTION('center_axis',(0.,0.,-1.));
#7237=DIRECTION('ref_axis',(1.,0.,0.));
#7238=DIRECTION('center_axis',(0.,0.,1.));
#7239=DIRECTION('ref_axis',(1.,0.,0.));
#7240=DIRECTION('center_axis',(0.,0.,1.));
#7241=DIRECTION('ref_axis',(1.,0.,0.));
#7242=DIRECTION('',(0.,0.,1.));
#7243=DIRECTION('center_axis',(0.,0.,1.));
#7244=DIRECTION('ref_axis',(-1.,7.6571373978539E-16,0.));
#7245=DIRECTION('center_axis',(0.,0.,1.));
#7246=DIRECTION('ref_axis',(1.,0.,0.));
#7247=DIRECTION('center_axis',(0.,0.,1.));
#7248=DIRECTION('ref_axis',(1.,0.,0.));
#7249=DIRECTION('',(0.,0.,-1.));
#7250=DIRECTION('center_axis',(0.,0.,1.));
#7251=DIRECTION('ref_axis',(1.,0.,0.));
#7252=DIRECTION('center_axis',(0.,0.,1.));
#7253=DIRECTION('ref_axis',(1.,0.,0.));
#7254=DIRECTION('center_axis',(0.,0.,-1.));
#7255=DIRECTION('ref_axis',(1.,0.,0.));
#7256=DIRECTION('',(0.,0.,-1.));
#7257=DIRECTION('center_axis',(0.,0.,1.));
#7258=DIRECTION('ref_axis',(1.,0.,0.));
#7259=DIRECTION('',(1.,0.,0.));
#7260=DIRECTION('center_axis',(0.,0.,-1.));
#7261=DIRECTION('ref_axis',(1.,0.,0.));
#7262=DIRECTION('',(-1.,0.,0.));
#7263=DIRECTION('center_axis',(0.,0.,-1.));
#7264=DIRECTION('ref_axis',(1.,0.,0.));
#7265=DIRECTION('center_axis',(0.,0.,-1.));
#7266=DIRECTION('ref_axis',(1.,0.,0.));
#7267=DIRECTION('center_axis',(0.,-1.,0.));
#7268=DIRECTION('ref_axis',(1.,0.,0.));
#7269=DIRECTION('',(0.,0.,-1.));
#7270=DIRECTION('center_axis',(0.,1.,0.));
#7271=DIRECTION('ref_axis',(-1.,0.,0.));
#7272=DIRECTION('',(0.,0.,1.));
#7273=DIRECTION('center_axis',(0.,0.,1.));
#7274=DIRECTION('ref_axis',(1.,0.,0.));
#7275=DIRECTION('',(0.,0.,-1.));
#7276=DIRECTION('center_axis',(0.,0.,-1.));
#7277=DIRECTION('ref_axis',(1.,0.,0.));
#7278=DIRECTION('center_axis',(0.,0.,1.));
#7279=DIRECTION('ref_axis',(1.,0.,0.));
#7280=DIRECTION('center_axis',(0.,0.,1.));
#7281=DIRECTION('ref_axis',(1.,0.,0.));
#7282=DIRECTION('',(0.,0.,-1.));
#7283=DIRECTION('center_axis',(0.,0.,1.));
#7284=DIRECTION('ref_axis',(1.,0.,0.));
#7285=DIRECTION('center_axis',(0.,0.,1.));
#7286=DIRECTION('ref_axis',(1.,0.,0.));
#7287=DIRECTION('center_axis',(0.,0.,1.));
#7288=DIRECTION('ref_axis',(1.,0.,0.));
#8652=CARTESIAN_POINT('',(0.,0.,0.));
#8653=CARTESIAN_POINT('Origin',(0.,0.,3.8));
#8654=CARTESIAN_POINT('',(-6.35,-7.77650717458569E-16,3.8));
#8655=CARTESIAN_POINT('Origin',(0.,0.,3.8));
#8656=CARTESIAN_POINT('',(-6.35,-7.77650717458569E-16,3.6));
#8657=CARTESIAN_POINT('',(-6.35,7.77650717458569E-16,3.8));
#8658=CARTESIAN_POINT('Origin',(0.,0.,3.6));
#8659=CARTESIAN_POINT('Origin',(0.,0.,3.8));
#8660=CARTESIAN_POINT('',(-6.85,-8.38883057415937E-16,3.8));
#8661=CARTESIAN_POINT('Origin',(0.,0.,3.8));
#8662=CARTESIAN_POINT('',(-6.85,-8.38883057415937E-16,3.6));
#8663=CARTESIAN_POINT('',(-6.85,8.38883057415937E-16,3.8));
#8664=CARTESIAN_POINT('Origin',(0.,0.,3.6));
#8665=CARTESIAN_POINT('Origin',(0.,0.,3.6));
#8666=CARTESIAN_POINT('Origin',(0.,0.,3.8));
#8667=CARTESIAN_POINT('',(-6.2,-7.59281015471359E-16,3.8));
#8668=CARTESIAN_POINT('Origin',(0.,0.,3.8));
#8669=CARTESIAN_POINT('Origin',(-7.4,0.,1.9));
#8670=CARTESIAN_POINT('',(-7.75,4.28626379701574E-17,3.8));
#8671=CARTESIAN_POINT('Origin',(-7.4,0.,3.8));
#8672=CARTESIAN_POINT('',(-7.75,4.28626379701574E-17,-2.22044604925031E-16));
#8673=CARTESIAN_POINT('',(-7.75,4.28626379701574E-17,1.9));
#8674=CARTESIAN_POINT('Origin',(-7.4,0.,0.));
#8675=CARTESIAN_POINT('Origin',(7.4,0.,1.9));
#8676=CARTESIAN_POINT('',(7.05,4.28626379701574E-17,3.8));
#8677=CARTESIAN_POINT('Origin',(7.4,0.,3.8));
#8678=CARTESIAN_POINT('',(7.05,4.28626379701574E-17,-2.22044604925031E-16));
#8679=CARTESIAN_POINT('',(7.05,4.28626379701574E-17,1.9));
#8680=CARTESIAN_POINT('Origin',(7.4,0.,0.));
#8681=CARTESIAN_POINT('Origin',(0.,7.4,1.9));
#8682=CARTESIAN_POINT('',(-0.35,7.4,3.8));
#8683=CARTESIAN_POINT('Origin',(0.,7.4,3.8));
#8684=CARTESIAN_POINT('',(-0.35,7.4,-2.22044604925031E-16));
#8685=CARTESIAN_POINT('',(-0.35,7.4,1.9));
#8686=CARTESIAN_POINT('Origin',(0.,7.4,0.));
#8687=CARTESIAN_POINT('Origin',(0.,-7.4,1.9));
#8688=CARTESIAN_POINT('',(-0.35,-7.4,3.8));
#8689=CARTESIAN_POINT('Origin',(0.,-7.4,3.8));
#8690=CARTESIAN_POINT('',(-0.35,-7.4,-2.22044604925031E-16));
#8691=CARTESIAN_POINT('',(-0.35,-7.4,1.9));
#8692=CARTESIAN_POINT('Origin',(0.,-7.4,0.));
#8693=CARTESIAN_POINT('Origin',(1.18660254037844,-1.85525588832577,3.2));
#8694=CARTESIAN_POINT('',(0.926794919243111,-2.00525588832577,3.2));
#8695=CARTESIAN_POINT('',(1.18660254037844,-1.85525588832577,3.2));
#8696=CARTESIAN_POINT('',(3.39330127018922,-0.58121778264911,3.2));
#8697=CARTESIAN_POINT('',(0.926794919243111,-2.00525588832577,3.8));
#8698=CARTESIAN_POINT('',(0.926794919243111,-2.00525588832577,3.2));
#8699=CARTESIAN_POINT('',(1.18660254037844,-1.85525588832577,3.8));
#8700=CARTESIAN_POINT('',(0.926794919243111,-2.00525588832577,3.8));
#8701=CARTESIAN_POINT('',(1.18660254037844,-1.85525588832577,3.2));
#8702=CARTESIAN_POINT('Origin',(3.69807621135331,-0.405255888325769,3.2));
#8703=CARTESIAN_POINT('',(3.39494366787712,-3.28936938489376,3.2));
#8704=CARTESIAN_POINT('Origin',(3.69807621135331,-0.405255888325769,3.2));
#8705=CARTESIAN_POINT('',(3.39494366787712,-3.28936938489376,3.8));
#8706=CARTESIAN_POINT('Origin',(3.69807621135331,-0.405255888325769,3.8));
#8707=CARTESIAN_POINT('',(3.39494366787712,-3.28936938489376,3.2));
#8708=CARTESIAN_POINT('Origin',(3.36358512889682,-3.58772595350424,3.2));
#8709=CARTESIAN_POINT('',(3.36358512889682,-3.58772595350424,3.2));
#8710=CARTESIAN_POINT('',(3.56447066879145,-1.6764277133635,3.2));
#8711=CARTESIAN_POINT('',(3.36358512889682,-3.58772595350424,3.8));
#8712=CARTESIAN_POINT('',(3.39494366787712,-3.28936938489376,3.8));
#8713=CARTESIAN_POINT('',(3.36358512889682,-3.58772595350424,3.2));
#8714=CARTESIAN_POINT('Origin',(3.69807621135331,-0.405255888325769,3.2));
#8715=CARTESIAN_POINT('Origin',(3.69807621135331,-0.405255888325769,3.2));
#8716=CARTESIAN_POINT('Origin',(3.69807621135331,-0.405255888325769,3.8));
#8717=CARTESIAN_POINT('Origin',(2.22154556813824,-2.75240702699307,3.8));
#8718=CARTESIAN_POINT('Origin',(-1.01339745962156,-1.95525588832576,3.2));
#8719=CARTESIAN_POINT('',(-1.27320508075689,-1.80525588832576,3.2));
#8720=CARTESIAN_POINT('',(-1.01339745962156,-1.95525588832576,3.2));
#8721=CARTESIAN_POINT('',(1.19330127018922,-3.22929399400242,3.2));
#8722=CARTESIAN_POINT('',(-1.27320508075689,-1.80525588832576,3.8));
#8723=CARTESIAN_POINT('',(-1.27320508075689,-1.80525588832576,3.2));
#8724=CARTESIAN_POINT('',(-1.01339745962156,-1.95525588832576,3.8));
#8725=CARTESIAN_POINT('',(-1.27320508075689,-1.80525588832576,3.8));
#8726=CARTESIAN_POINT('',(-1.01339745962156,-1.95525588832576,3.2));
#8727=CARTESIAN_POINT('Origin',(1.49807621135331,-3.40525588832577,3.2));
#8728=CARTESIAN_POINT('',(-1.15120561581023,-4.58479215324559,3.2));
#8729=CARTESIAN_POINT('Origin',(1.49807621135331,-3.40525588832577,3.2));
#8730=CARTESIAN_POINT('',(-1.15120561581023,-4.58479215324559,3.8));
#8731=CARTESIAN_POINT('Origin',(1.49807621135331,-3.40525588832577,3.8));
#8732=CARTESIAN_POINT('',(-1.15120561581023,-4.58479215324559,3.2));
#8733=CARTESIAN_POINT('Origin',(-1.42526925310301,-4.70681314616832,3.2));
#8734=CARTESIAN_POINT('',(-1.42526925310301,-4.70681314616832,3.2));
#8735=CARTESIAN_POINT('',(2.54762774811539,-2.93796543744964,3.2));
#8736=CARTESIAN_POINT('',(-1.42526925310301,-4.70681314616832,3.8));
#8737=CARTESIAN_POINT('',(-1.15120561581023,-4.58479215324559,3.8));
#8738=CARTESIAN_POINT('',(-1.42526925310301,-4.70681314616832,3.2));
#8739=CARTESIAN_POINT('Origin',(1.49807621135331,-3.40525588832577,3.2));
#8740=CARTESIAN_POINT('Origin',(1.49807621135331,-3.40525588832577,3.2));
#8741=CARTESIAN_POINT('Origin',(1.49807621135331,-3.40525588832577,3.8));
#8742=CARTESIAN_POINT('Origin',(-1.27288162286168,-3.30011841116898,3.8));
#8743=CARTESIAN_POINT('Origin',(-2.2,-0.0999999999999998,3.2));
#8744=CARTESIAN_POINT('',(-2.2,0.2,3.2));
#8745=CARTESIAN_POINT('',(-2.2,-0.0999999999999998,3.2));
#8746=CARTESIAN_POINT('',(-2.2,-0.0499999999999992,3.2));
#8747=CARTESIAN_POINT('',(-2.2,0.2,3.8));
#8748=CARTESIAN_POINT('',(-2.2,0.2,3.2));
#8749=CARTESIAN_POINT('',(-2.2,-0.0999999999999998,3.8));
#8750=CARTESIAN_POINT('',(-2.2,0.2,3.8));
#8751=CARTESIAN_POINT('',(-2.2,-0.0999999999999998,3.2));
#8752=CARTESIAN_POINT('Origin',(-2.2,-3.,3.2));
#8753=CARTESIAN_POINT('',(-4.54614928368735,-1.29542276835183,3.2));
#8754=CARTESIAN_POINT('Origin',(-2.2,-3.,3.2));
#8755=CARTESIAN_POINT('',(-4.54614928368735,-1.29542276835183,3.8));
#8756=CARTESIAN_POINT('Origin',(-2.2,-3.,3.8));
#8757=CARTESIAN_POINT('',(-4.54614928368735,-1.29542276835183,3.2));
#8758=CARTESIAN_POINT('Origin',(-4.78885438199983,-1.11908719266409,3.2));
#8759=CARTESIAN_POINT('',(-4.78885438199983,-1.11908719266409,3.2));
#8760=CARTESIAN_POINT('',(-1.52423473975264,-3.49097220051832,3.2));
#8761=CARTESIAN_POINT('',(-4.78885438199983,-1.11908719266409,3.8));
#8762=CARTESIAN_POINT('',(-4.54614928368735,-1.29542276835183,3.8));
#8763=CARTESIAN_POINT('',(-4.78885438199983,-1.11908719266409,3.2));
#8764=CARTESIAN_POINT('Origin',(-2.2,-3.,3.2));
#8765=CARTESIAN_POINT('Origin',(-2.2,-3.,3.2));
#8766=CARTESIAN_POINT('Origin',(-2.2,-3.,3.8));
#8767=CARTESIAN_POINT('Origin',(-3.49442719099992,-0.547711384175914,3.8));
#8768=CARTESIAN_POINT('Origin',(-1.18660254037844,1.85525588832577,3.2));
#8769=CARTESIAN_POINT('',(-0.926794919243112,2.00525588832577,3.2));
#8770=CARTESIAN_POINT('',(-1.18660254037844,1.85525588832577,3.2));
#8771=CARTESIAN_POINT('',(1.10669872981078,3.17929399400242,3.2));
#8772=CARTESIAN_POINT('',(-0.926794919243112,2.00525588832577,3.8));
#8773=CARTESIAN_POINT('',(-0.926794919243112,2.00525588832577,3.2));
#8774=CARTESIAN_POINT('',(-1.18660254037844,1.85525588832577,3.8));
#8775=CARTESIAN_POINT('',(-0.926794919243112,2.00525588832577,3.8));
#8776=CARTESIAN_POINT('',(-1.18660254037844,1.85525588832577,3.2));
#8777=CARTESIAN_POINT('Origin',(-3.69807621135331,0.405255888325767,3.2));
#8778=CARTESIAN_POINT('',(-3.39494366787712,3.28936938489376,3.2));
#8779=CARTESIAN_POINT('Origin',(-3.69807621135331,0.405255888325767,3.2));
#8780=CARTESIAN_POINT('',(-3.39494366787712,3.28936938489376,3.8));
#8781=CARTESIAN_POINT('Origin',(-3.69807621135331,0.405255888325767,3.8));
#8782=CARTESIAN_POINT('',(-3.39494366787712,3.28936938489376,3.2));
#8783=CARTESIAN_POINT('Origin',(-3.36358512889682,3.58772595350424,3.2));
#8784=CARTESIAN_POINT('',(-3.36358512889682,3.58772595350424,3.2));
#8785=CARTESIAN_POINT('',(-3.49891347099287,2.30016278581678,3.2));
#8786=CARTESIAN_POINT('',(-3.36358512889682,3.58772595350424,3.8));
#8787=CARTESIAN_POINT('',(-3.39494366787712,3.28936938489376,3.8));
#8788=CARTESIAN_POINT('',(-3.36358512889682,3.58772595350424,3.2));
#8789=CARTESIAN_POINT('Origin',(-3.69807621135332,0.405255888325766,3.2));
#8790=CARTESIAN_POINT('Origin',(-3.69807621135332,0.405255888325766,3.2));
#8791=CARTESIAN_POINT('Origin',(-3.69807621135332,0.405255888325766,3.8));
#8792=CARTESIAN_POINT('Origin',(-2.22154556813824,2.75240702699307,3.8));
#8793=CARTESIAN_POINT('Origin',(1.01339745962156,1.95525588832577,3.2));
#8794=CARTESIAN_POINT('',(1.27320508075689,1.80525588832577,3.2));
#8795=CARTESIAN_POINT('',(1.01339745962156,1.95525588832577,3.2));
#8796=CARTESIAN_POINT('',(3.30669872981078,0.631217782649107,3.2));
#8797=CARTESIAN_POINT('',(1.27320508075689,1.80525588832577,3.8));
#8798=CARTESIAN_POINT('',(1.27320508075689,1.80525588832577,3.2));
#8799=CARTESIAN_POINT('',(1.01339745962156,1.95525588832577,3.8));
#8800=CARTESIAN_POINT('',(1.27320508075689,1.80525588832577,3.8));
#8801=CARTESIAN_POINT('',(1.01339745962156,1.95525588832577,3.2));
#8802=CARTESIAN_POINT('Origin',(-1.49807621135331,3.40525588832576,3.2));
#8803=CARTESIAN_POINT('',(1.15120561581023,4.58479215324559,3.2));
#8804=CARTESIAN_POINT('Origin',(-1.49807621135331,3.40525588832576,3.2));
#8805=CARTESIAN_POINT('',(1.15120561581023,4.58479215324559,3.8));
#8806=CARTESIAN_POINT('Origin',(-1.49807621135331,3.40525588832576,3.8));
#8807=CARTESIAN_POINT('',(1.15120561581023,4.58479215324559,3.2));
#8808=CARTESIAN_POINT('Origin',(1.42526925310301,4.70681314616832,3.2));
#8809=CARTESIAN_POINT('',(1.42526925310301,4.70681314616833,3.2));
#8810=CARTESIAN_POINT('',(2.45976407096119,5.16739991388182,3.2));
#8811=CARTESIAN_POINT('',(1.42526925310301,4.70681314616833,3.8));
#8812=CARTESIAN_POINT('',(1.15120561581023,4.58479215324559,3.8));
#8813=CARTESIAN_POINT('',(1.42526925310301,4.70681314616833,3.2));
#8814=CARTESIAN_POINT('Origin',(-1.49807621135332,3.40525588832576,3.2));
#8815=CARTESIAN_POINT('Origin',(-1.49807621135332,3.40525588832576,3.2));
#8816=CARTESIAN_POINT('Origin',(-1.49807621135332,3.40525588832576,3.8));
#8817=CARTESIAN_POINT('Origin',(1.27288162286168,3.30011841116898,3.8));
#8818=CARTESIAN_POINT('Origin',(2.2,0.1,3.2));
#8819=CARTESIAN_POINT('',(2.2,-0.2,3.2));
#8820=CARTESIAN_POINT('',(2.2,0.1,3.2));
#8821=CARTESIAN_POINT('',(2.2,0.05,3.2));
#8822=CARTESIAN_POINT('',(2.2,-0.2,3.8));
#8823=CARTESIAN_POINT('',(2.2,-0.2,3.2));
#8824=CARTESIAN_POINT('',(2.2,0.1,3.8));
#8825=CARTESIAN_POINT('',(2.2,-0.2,3.8));
#8826=CARTESIAN_POINT('',(2.2,0.1,3.2));
#8827=CARTESIAN_POINT('Origin',(2.2,3.,3.2));
#8828=CARTESIAN_POINT('',(4.54614928368735,1.29542276835183,3.2));
#8829=CARTESIAN_POINT('Origin',(2.2,3.,3.2));
#8830=CARTESIAN_POINT('',(4.54614928368735,1.29542276835183,3.8));
#8831=CARTESIAN_POINT('Origin',(2.2,3.,3.8));
#8832=CARTESIAN_POINT('',(4.54614928368735,1.29542276835183,3.2));
#8833=CARTESIAN_POINT('Origin',(4.78885438199983,1.11908719266409,3.2));
#8834=CARTESIAN_POINT('',(4.78885438199983,1.11908719266409,3.2));
#8835=CARTESIAN_POINT('',(5.45128572287748,0.637802651632858,3.2));
#8836=CARTESIAN_POINT('',(4.78885438199983,1.11908719266409,3.8));
#8837=CARTESIAN_POINT('',(4.54614928368735,1.29542276835183,3.8));
#8838=CARTESIAN_POINT('',(4.78885438199983,1.11908719266409,3.2));
#8839=CARTESIAN_POINT('Origin',(2.2,3.,3.2));
#8840=CARTESIAN_POINT('Origin',(2.2,3.,3.2));
#8841=CARTESIAN_POINT('Origin',(2.2,3.,3.8));
#8842=CARTESIAN_POINT('Origin',(3.49442719099992,0.547711384175914,3.8));
#8843=CARTESIAN_POINT('Origin',(-2.85358983848623,-5.74256258422041,2.8));
#8844=CARTESIAN_POINT('',(-2.54668506678411,-5.21098792654702,3.2));
#8845=CARTESIAN_POINT('',(-2.54668506678411,-5.21098792654702,2.8));
#8846=CARTESIAN_POINT('',(-2.54668506678411,-5.21098792654702,2.8));
#8847=CARTESIAN_POINT('',(-2.74713149813783,-5.55817132984753,3.2));
#8848=CARTESIAN_POINT('',(-2.85358983848623,-5.74256258422041,3.2));
#8849=CARTESIAN_POINT('',(-2.74713149813783,-5.55817132984753,2.8));
#8850=CARTESIAN_POINT('',(-2.74713149813783,-5.55817132984753,0.));
#8851=CARTESIAN_POINT('',(-2.85358983848623,-5.74256258422041,2.8));
#8852=CARTESIAN_POINT('Origin',(-3.14641016151378,-4.64974226119285,2.8));
#8853=CARTESIAN_POINT('',(-3.23950538981167,-4.81098792654702,2.8));
#8854=CARTESIAN_POINT('',(-3.23950538981167,-4.81098792654702,3.2));
#8855=CARTESIAN_POINT('',(-3.23950538981167,-4.81098792654702,2.8));
#8856=CARTESIAN_POINT('',(-3.43995182116538,-5.15817132984752,2.8));
#8857=CARTESIAN_POINT('',(-3.14641016151378,-4.64974226119285,2.8));
#8858=CARTESIAN_POINT('',(-3.43995182116538,-5.15817132984752,3.2));
#8859=CARTESIAN_POINT('',(-3.43995182116538,-5.15817132984752,0.));
#8860=CARTESIAN_POINT('',(-3.14641016151378,-4.64974226119285,3.2));
#8861=CARTESIAN_POINT('Origin',(-3.54641016151377,5.34256258422041,2.8));
#8862=CARTESIAN_POINT('',(-3.23950538981166,4.81098792654702,3.2));
#8863=CARTESIAN_POINT('',(-3.23950538981166,4.81098792654702,2.8));
#8864=CARTESIAN_POINT('',(-3.23950538981166,4.81098792654702,2.8));
#8865=CARTESIAN_POINT('',(-3.43995182116538,5.15817132984753,3.2));
#8866=CARTESIAN_POINT('',(-3.54641016151377,5.34256258422041,3.2));
#8867=CARTESIAN_POINT('',(-3.43995182116538,5.15817132984753,2.8));
#8868=CARTESIAN_POINT('',(-3.43995182116538,5.15817132984753,0.));
#8869=CARTESIAN_POINT('',(-3.54641016151377,5.34256258422041,2.8));
#8870=CARTESIAN_POINT('Origin',(-2.45358983848622,5.04974226119286,2.8));
#8871=CARTESIAN_POINT('',(-2.54668506678411,5.21098792654702,2.8));
#8872=CARTESIAN_POINT('',(-2.54668506678411,5.21098792654702,3.2));
#8873=CARTESIAN_POINT('',(-2.54668506678411,5.21098792654702,2.8));
#8874=CARTESIAN_POINT('',(-2.74713149813783,5.55817132984753,2.8));
#8875=CARTESIAN_POINT('',(-2.45358983848622,5.04974226119286,2.8));
#8876=CARTESIAN_POINT('',(-2.74713149813783,5.55817132984753,3.2));
#8877=CARTESIAN_POINT('',(-2.74713149813783,5.55817132984753,0.));
#8878=CARTESIAN_POINT('',(-2.45358983848622,5.04974226119286,3.2));
#8879=CARTESIAN_POINT('Origin',(6.,0.,2.8));
#8880=CARTESIAN_POINT('Origin',(0.,0.,2.8));
#8881=CARTESIAN_POINT('Origin',(0.,0.,2.8));
#8882=CARTESIAN_POINT('',(5.78619045659577,0.4,2.8));
#8883=CARTESIAN_POINT('Origin',(0.,0.,2.8));
#8884=CARTESIAN_POINT('',(6.18708331930321,0.4,2.8));
#8885=CARTESIAN_POINT('',(6.4,0.4,2.8));
#8886=CARTESIAN_POINT('',(6.18708331930321,-0.4,2.8));
#8887=CARTESIAN_POINT('Origin',(0.,0.,2.8));
#8888=CARTESIAN_POINT('',(5.78619045659577,-0.4,2.8));
#8889=CARTESIAN_POINT('',(5.6,-0.4,2.8));
#8890=CARTESIAN_POINT('Origin',(0.,0.,2.8));
#8891=CARTESIAN_POINT('Origin',(0.,0.,2.8));
#8892=CARTESIAN_POINT('',(-1.7,-2.0818995585505E-16,2.8));
#8893=CARTESIAN_POINT('Origin',(0.,0.,2.8));
#8894=CARTESIAN_POINT('Origin',(0.,0.,2.8));
#8895=CARTESIAN_POINT('',(5.78619045659577,0.4,3.2));
#8896=CARTESIAN_POINT('Origin',(0.,0.,3.2));
#8897=CARTESIAN_POINT('',(5.78619045659577,0.4,2.8));
#8898=CARTESIAN_POINT('Origin',(0.,0.,2.8));
#8899=CARTESIAN_POINT('Origin',(0.,0.,3.2));
#8900=CARTESIAN_POINT('Origin',(0.,0.,2.8));
#8901=CARTESIAN_POINT('',(5.78619045659577,-0.4,3.2));
#8902=CARTESIAN_POINT('',(5.78619045659577,-0.4,2.8));
#8903=CARTESIAN_POINT('Origin',(0.,0.,3.2));
#8904=CARTESIAN_POINT('Origin',(0.,0.,2.8));
#8905=CARTESIAN_POINT('',(-1.7,-2.0818995585505E-16,3.2));
#8906=CARTESIAN_POINT('Origin',(0.,0.,3.2));
#8907=CARTESIAN_POINT('',(-1.7,-2.0818995585505E-16,2.8));
#8908=CARTESIAN_POINT('Origin',(6.,0.,3.2));
#8909=CARTESIAN_POINT('',(6.18708331930321,-0.4,3.2));
#8910=CARTESIAN_POINT('',(5.6,-0.4,3.2));
#8911=CARTESIAN_POINT('',(6.18708331930321,0.4,3.2));
#8912=CARTESIAN_POINT('Origin',(0.,0.,3.2));
#8913=CARTESIAN_POINT('',(6.4,0.4,3.2));
#8914=CARTESIAN_POINT('Origin',(0.,0.,3.2));
#8915=CARTESIAN_POINT('Origin',(0.,0.,3.2));
#8916=CARTESIAN_POINT('Origin',(5.6,-0.4,2.8));
#8917=CARTESIAN_POINT('',(6.18708331930321,-0.4,0.));
#8918=CARTESIAN_POINT('Origin',(6.4,0.4,2.8));
#8919=CARTESIAN_POINT('',(6.18708331930321,0.4,0.));
#8920=CARTESIAN_POINT('Origin',(0.,0.,0.));
#8921=CARTESIAN_POINT('',(-6.2,-7.59281015471359E-16,0.));
#8922=CARTESIAN_POINT('',(-6.2,-7.59281015471359E-16,0.));
#8923=CARTESIAN_POINT('Origin',(0.,0.,0.));
#8924=CARTESIAN_POINT('Origin',(0.,0.,0.));
#8925=CARTESIAN_POINT('',(-8.2,-1.00421037530083E-15,3.8));
#8926=CARTESIAN_POINT('Origin',(0.,0.,3.8));
#8927=CARTESIAN_POINT('',(-8.2,-1.00421037530083E-15,0.));
#8928=CARTESIAN_POINT('',(-8.2,-1.00421037530083E-15,0.));
#8929=CARTESIAN_POINT('Origin',(0.,0.,0.));
#8930=CARTESIAN_POINT('Origin',(0.,0.,3.8));
#8931=CARTESIAN_POINT('Origin',(0.,0.,0.));
#16647=UNCERTAINTY_MEASURE_WITH_UNIT(LENGTH_MEASURE(0.001),#16688,
'DISTANCE_ACCURACY_VALUE',
'Maximum model space distance between geometric entities at asserted c
onnectivities');
#16666=UNCERTAINTY_MEASURE_WITH_UNIT(LENGTH_MEASURE(0.001),#16688,
'DISTANCE_ACCURACY_VALUE',
'Maximum model space distance between geometric entities at asserted c
onnectivities');
#16668=(
GEOMETRIC_REPRESENTATION_CONTEXT(3)
GLOBAL_UNCERTAINTY_ASSIGNED_CONTEXT((#16647))
GLOBAL_UNIT_ASSIGNED_CONTEXT((#16688,#16690,#16691))
REPRESENTATION_CONTEXT('','3D')
);
#16687=(
GEOMETRIC_REPRESENTATION_CONTEXT(3)
GLOBAL_UNCERTAINTY_ASSIGNED_CONTEXT((#16666))
GLOBAL_UNIT_ASSIGNED_CONTEXT((#16688,#16690,#16691))
REPRESENTATION_CONTEXT('','3D')
);
#16688=(
LENGTH_UNIT()
NAMED_UNIT(*)
SI_UNIT(.CENTI.,.METRE.)
);
#16690=(
NAMED_UNIT(*)
PLANE_ANGLE_UNIT()
SI_UNIT($,.RADIAN.)
);
#16691=(
NAMED_UNIT(*)
SI_UNIT($,.STERADIAN.)
SOLID_ANGLE_UNIT()
);
#16693=SHAPE_DEFINITION_REPRESENTATION(#16713,#16764);
#16713=PRODUCT_DEFINITION_SHAPE('',$,#16785);
#16764=SHAPE_REPRESENTATION('',(#6342),#16668);
#16783=PRODUCT_DEFINITION_CONTEXT('part definition',#16845,'design');
#16785=PRODUCT_DEFINITION('Stage casing','Stage casing',#16805,#16783);
#16805=PRODUCT_DEFINITION_FORMATION('',$,#16848);
#16845=APPLICATION_CONTEXT(
'Core Data for Automotive Mechanical Design Process');
#16846=PRODUCT_CONTEXT('part definition',#16845,'mechanical');
#16848=PRODUCT('Stage casing','Stage casing',$,(#16846));
#16868=PRESENTATION_STYLE_ASSIGNMENT((#16883));
#16883=SURFACE_STYLE_USAGE(.BOTH.,#16898);
#16898=SURFACE_SIDE_STYLE('',(#16913));
#16913=SURFACE_STYLE_FILL_AREA(#16928);
#16928=FILL_AREA_STYLE('Dark blue',(#16943));
#16943=FILL_AREA_STYLE_COLOUR('Dark blue',#16958);
#16958=COLOUR_RGB('Dark blue',0.0901960784313725,0.270588235294118,0.513725490196078);
ENDSEC;
END-ISO-10303-21;
